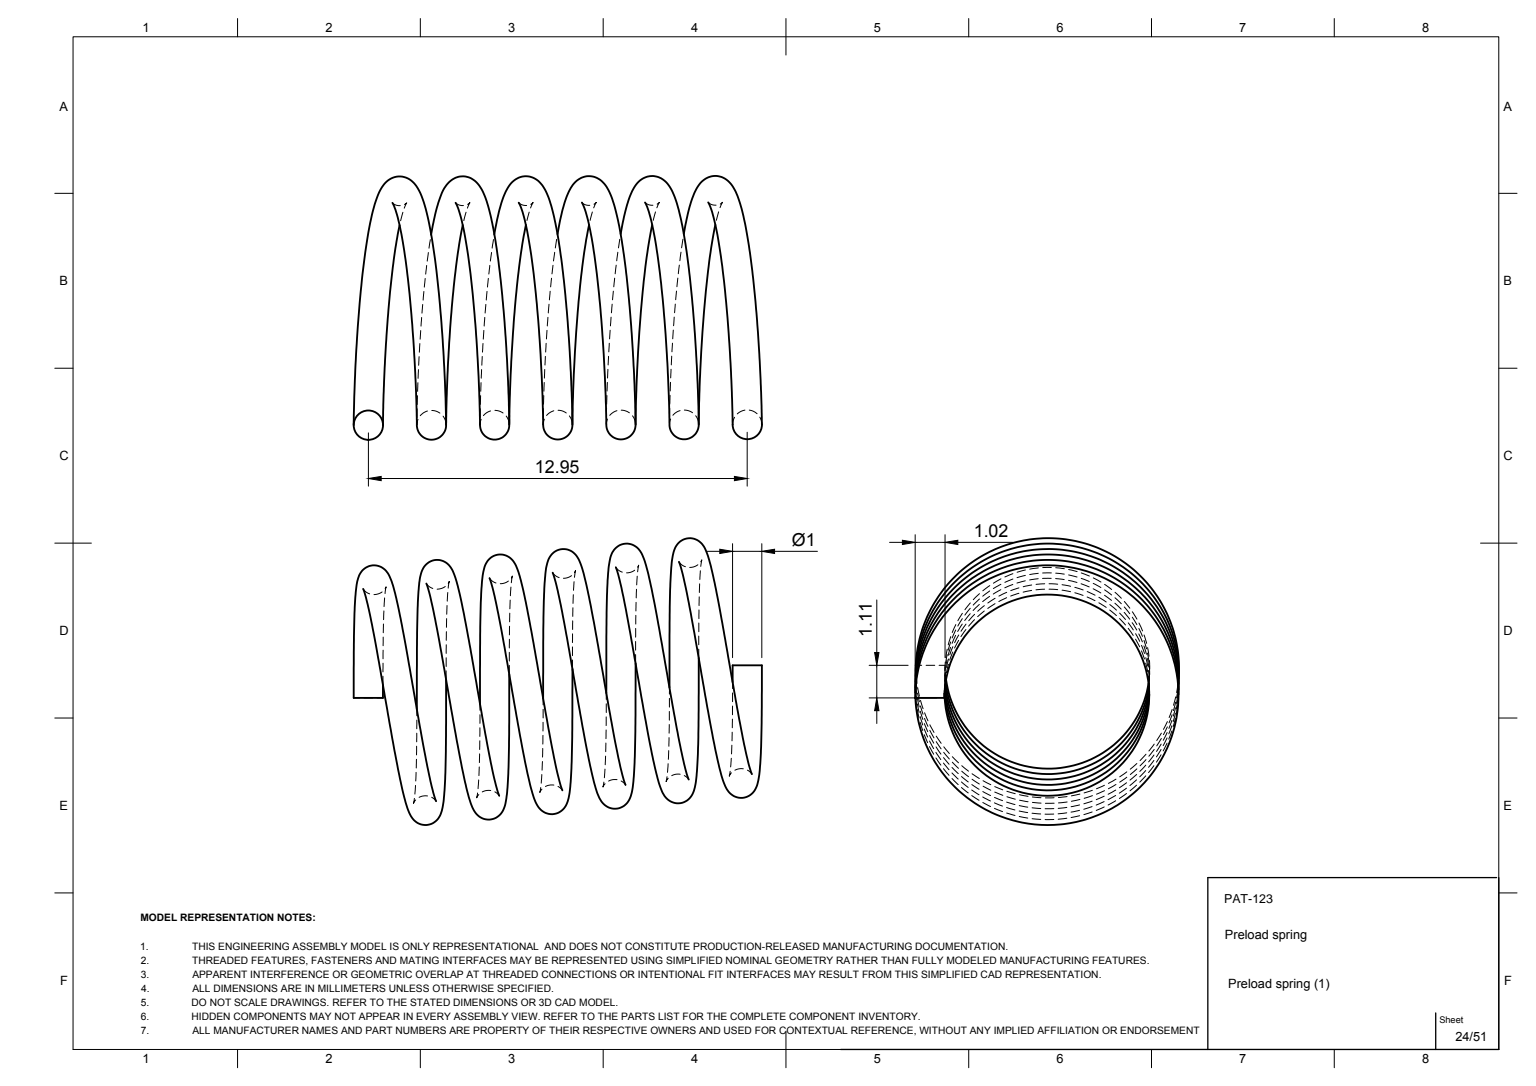
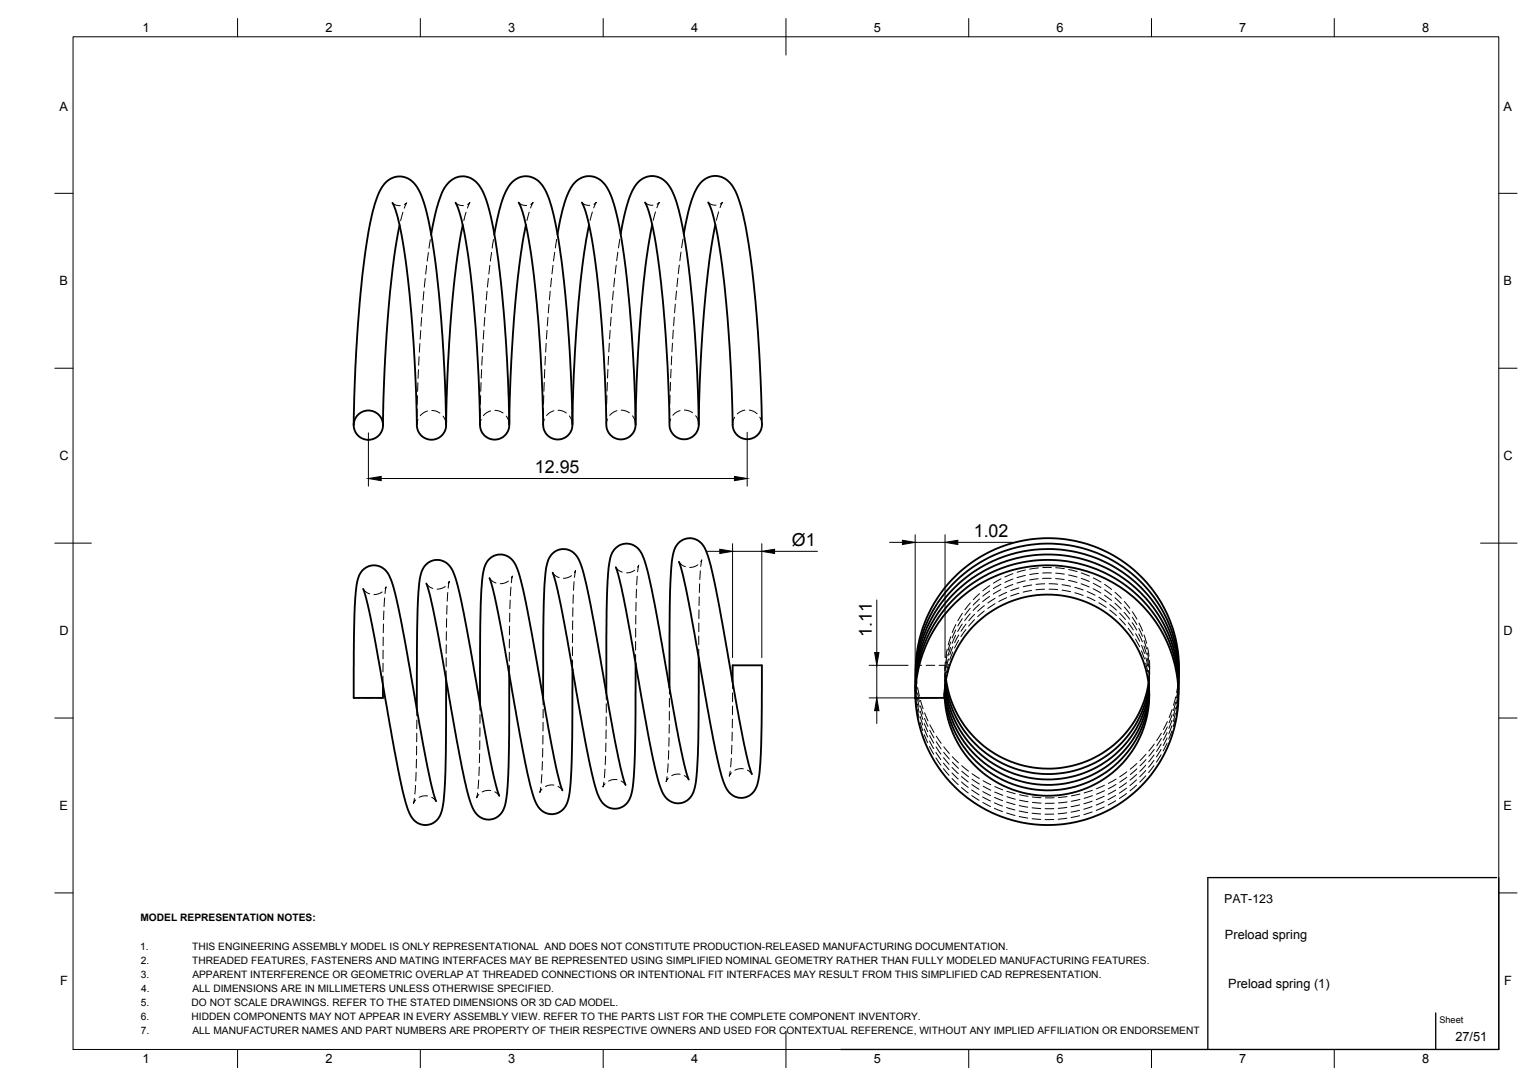
ISO-10303-21;
HEADER;
/* Generated by software containing ST-Developer
 * from STEP Tools, Inc. (www.steptools.com) 
 */

FILE_DESCRIPTION(
/* description */ ('Worm-less right-angle friction wheel drive'),
/* implementation_level */ '2;1');

FILE_NAME(
/* name */ 'Preload spring.step',
/* time_stamp */ '2026-10-28T03:22:36-07:00',
/* author */ (''),
/* organization */ (''),
/* preprocessor_version */ 'ST-DEVELOPER v20.2',
/* originating_system */ 'Autodesk Translation Framework v15.17.0.0',
/* authorisation */ '');

FILE_SCHEMA (('AUTOMOTIVE_DESIGN { 1 0 10303 214 3 1 1 }'));
ENDSEC;

DATA;
#10=MECHANICAL_DESIGN_GEOMETRIC_PRESENTATION_REPRESENTATION('',(#630),#17046);
#481=B_SPLINE_CURVE_WITH_KNOTS('',3,(#14322,#14323,#14324,#14325,#14326,
#14327,#14328,#14329,#14330,#14331,#14332,#14333,#14334,#14335,#14336,#14337,
#14338,#14339,#14340,#14341,#14342,#14343,#14344,#14345,#14346,#14347,#14348,
#14349,#14350,#14351,#14352,#14353,#14354,#14355,#14356,#14357,#14358,#14359,
#14360,#14361,#14362,#14363,#14364,#14365,#14366,#14367,#14368,#14369,#14370,
#14371,#14372,#14373,#14374,#14375,#14376,#14377,#14378,#14379,#14380,#14381,
#14382,#14383,#14384,#14385,#14386,#14387,#14388,#14389,#14390,#14391,#14392,
#14393,#14394,#14395,#14396,#14397,#14398,#14399,#14400,#14401,#14402,#14403,
#14404),.UNSPECIFIED.,.F.,.F.,(4,1,1,1,1,1,1,1,1,1,1,1,1,1,1,1,1,1,1,1,
1,1,1,1,1,1,1,1,1,1,1,1,1,1,1,1,1,1,1,1,1,1,1,1,1,1,1,1,1,1,1,1,1,1,1,1,
1,1,1,1,1,1,1,1,1,1,1,1,1,1,1,1,1,1,1,1,1,1,1,1,4),(0.,0.00892857142857143,
0.0178571428571429,0.0357142857142857,0.0535714285714286,0.0714285714285714,
0.0892857142857143,0.107142857142857,0.125,0.142857142857143,0.158730158730159,
0.174603174603175,0.19047619047619,0.202380952380952,0.214285714285714,
0.226190476190476,0.238095238095238,0.25,0.261904761904762,0.273809523809524,
0.285714285714286,0.297619047619048,0.30952380952381,0.321428571428571,
0.333333333333333,0.349206349206349,0.365079365079365,0.376984126984127,
0.380952380952381,0.392857142857143,0.404761904761905,0.416666666666667,
0.428571428571429,0.446428571428571,0.464285714285714,0.476190476190476,
0.488095238095238,0.5,0.508928571428571,0.517857142857143,0.526785714285714,
0.535714285714286,0.553571428571429,0.571428571428571,0.589285714285714,
0.607142857142857,0.625,0.633928571428571,0.642857142857143,0.654761904761905,
0.666666666666667,0.678571428571428,0.6875,0.696428571428571,0.705357142857143,
0.714285714285714,0.726190476190476,0.738095238095238,0.75,0.761904761904762,
0.773809523809524,0.785714285714286,0.791666666666667,0.797619047619047,
0.803571428571428,0.809523809523809,0.821428571428571,0.833333333333333,
0.845238095238095,0.857142857142857,0.866071428571429,0.875,0.883928571428571,
0.892857142857143,0.910714285714286,0.928571428571429,0.946428571428571,
0.964285714285714,0.982142857142857,0.991071428571429,1.),.UNSPECIFIED.);
#515=B_SPLINE_SURFACE_WITH_KNOTS('',3,3,((#13489,#13490,#13491,#13492,#13493,
#13494,#13495,#13496,#13497,#13498,#13499,#13500,#13501,#13502,#13503,#13504,
#13505,#13506,#13507,#13508,#13509,#13510,#13511,#13512,#13513,#13514,#13515,
#13516,#13517,#13518,#13519,#13520,#13521,#13522,#13523,#13524,#13525,#13526,
#13527,#13528,#13529,#13530,#13531,#13532,#13533,#13534,#13535,#13536,#13537,
#13538,#13539,#13540,#13541,#13542,#13543,#13544,#13545,#13546,#13547,#13548,
#13549,#13550,#13551,#13552,#13553,#13554,#13555,#13556,#13557,#13558,#13559,
#13560,#13561,#13562,#13563,#13564,#13565,#13566,#13567,#13568,#13569,#13570,
#13571),(#13572,#13573,#13574,#13575,#13576,#13577,#13578,#13579,#13580,
#13581,#13582,#13583,#13584,#13585,#13586,#13587,#13588,#13589,#13590,#13591,
#13592,#13593,#13594,#13595,#13596,#13597,#13598,#13599,#13600,#13601,#13602,
#13603,#13604,#13605,#13606,#13607,#13608,#13609,#13610,#13611,#13612,#13613,
#13614,#13615,#13616,#13617,#13618,#13619,#13620,#13621,#13622,#13623,#13624,
#13625,#13626,#13627,#13628,#13629,#13630,#13631,#13632,#13633,#13634,#13635,
#13636,#13637,#13638,#13639,#13640,#13641,#13642,#13643,#13644,#13645,#13646,
#13647,#13648,#13649,#13650,#13651,#13652,#13653,#13654),(#13655,#13656,
#13657,#13658,#13659,#13660,#13661,#13662,#13663,#13664,#13665,#13666,#13667,
#13668,#13669,#13670,#13671,#13672,#13673,#13674,#13675,#13676,#13677,#13678,
#13679,#13680,#13681,#13682,#13683,#13684,#13685,#13686,#13687,#13688,#13689,
#13690,#13691,#13692,#13693,#13694,#13695,#13696,#13697,#13698,#13699,#13700,
#13701,#13702,#13703,#13704,#13705,#13706,#13707,#13708,#13709,#13710,#13711,
#13712,#13713,#13714,#13715,#13716,#13717,#13718,#13719,#13720,#13721,#13722,
#13723,#13724,#13725,#13726,#13727,#13728,#13729,#13730,#13731,#13732,#13733,
#13734,#13735,#13736,#13737),(#13738,#13739,#13740,#13741,#13742,#13743,
#13744,#13745,#13746,#13747,#13748,#13749,#13750,#13751,#13752,#13753,#13754,
#13755,#13756,#13757,#13758,#13759,#13760,#13761,#13762,#13763,#13764,#13765,
#13766,#13767,#13768,#13769,#13770,#13771,#13772,#13773,#13774,#13775,#13776,
#13777,#13778,#13779,#13780,#13781,#13782,#13783,#13784,#13785,#13786,#13787,
#13788,#13789,#13790,#13791,#13792,#13793,#13794,#13795,#13796,#13797,#13798,
#13799,#13800,#13801,#13802,#13803,#13804,#13805,#13806,#13807,#13808,#13809,
#13810,#13811,#13812,#13813,#13814,#13815,#13816,#13817,#13818,#13819,#13820),
(#13821,#13822,#13823,#13824,#13825,#13826,#13827,#13828,#13829,#13830,
#13831,#13832,#13833,#13834,#13835,#13836,#13837,#13838,#13839,#13840,#13841,
#13842,#13843,#13844,#13845,#13846,#13847,#13848,#13849,#13850,#13851,#13852,
#13853,#13854,#13855,#13856,#13857,#13858,#13859,#13860,#13861,#13862,#13863,
#13864,#13865,#13866,#13867,#13868,#13869,#13870,#13871,#13872,#13873,#13874,
#13875,#13876,#13877,#13878,#13879,#13880,#13881,#13882,#13883,#13884,#13885,
#13886,#13887,#13888,#13889,#13890,#13891,#13892,#13893,#13894,#13895,#13896,
#13897,#13898,#13899,#13900,#13901,#13902,#13903),(#13904,#13905,#13906,
#13907,#13908,#13909,#13910,#13911,#13912,#13913,#13914,#13915,#13916,#13917,
#13918,#13919,#13920,#13921,#13922,#13923,#13924,#13925,#13926,#13927,#13928,
#13929,#13930,#13931,#13932,#13933,#13934,#13935,#13936,#13937,#13938,#13939,
#13940,#13941,#13942,#13943,#13944,#13945,#13946,#13947,#13948,#13949,#13950,
#13951,#13952,#13953,#13954,#13955,#13956,#13957,#13958,#13959,#13960,#13961,
#13962,#13963,#13964,#13965,#13966,#13967,#13968,#13969,#13970,#13971,#13972,
#13973,#13974,#13975,#13976,#13977,#13978,#13979,#13980,#13981,#13982,#13983,
#13984,#13985,#13986),(#13987,#13988,#13989,#13990,#13991,#13992,#13993,
#13994,#13995,#13996,#13997,#13998,#13999,#14000,#14001,#14002,#14003,#14004,
#14005,#14006,#14007,#14008,#14009,#14010,#14011,#14012,#14013,#14014,#14015,
#14016,#14017,#14018,#14019,#14020,#14021,#14022,#14023,#14024,#14025,#14026,
#14027,#14028,#14029,#14030,#14031,#14032,#14033,#14034,#14035,#14036,#14037,
#14038,#14039,#14040,#14041,#14042,#14043,#14044,#14045,#14046,#14047,#14048,
#14049,#14050,#14051,#14052,#14053,#14054,#14055,#14056,#14057,#14058,#14059,
#14060,#14061,#14062,#14063,#14064,#14065,#14066,#14067,#14068,#14069),
(#14070,#14071,#14072,#14073,#14074,#14075,#14076,#14077,#14078,#14079,
#14080,#14081,#14082,#14083,#14084,#14085,#14086,#14087,#14088,#14089,#14090,
#14091,#14092,#14093,#14094,#14095,#14096,#14097,#14098,#14099,#14100,#14101,
#14102,#14103,#14104,#14105,#14106,#14107,#14108,#14109,#14110,#14111,#14112,
#14113,#14114,#14115,#14116,#14117,#14118,#14119,#14120,#14121,#14122,#14123,
#14124,#14125,#14126,#14127,#14128,#14129,#14130,#14131,#14132,#14133,#14134,
#14135,#14136,#14137,#14138,#14139,#14140,#14141,#14142,#14143,#14144,#14145,
#14146,#14147,#14148,#14149,#14150,#14151,#14152),(#14153,#14154,#14155,
#14156,#14157,#14158,#14159,#14160,#14161,#14162,#14163,#14164,#14165,#14166,
#14167,#14168,#14169,#14170,#14171,#14172,#14173,#14174,#14175,#14176,#14177,
#14178,#14179,#14180,#14181,#14182,#14183,#14184,#14185,#14186,#14187,#14188,
#14189,#14190,#14191,#14192,#14193,#14194,#14195,#14196,#14197,#14198,#14199,
#14200,#14201,#14202,#14203,#14204,#14205,#14206,#14207,#14208,#14209,#14210,
#14211,#14212,#14213,#14214,#14215,#14216,#14217,#14218,#14219,#14220,#14221,
#14222,#14223,#14224,#14225,#14226,#14227,#14228,#14229,#14230,#14231,#14232,
#14233,#14234,#14235),(#14236,#14237,#14238,#14239,#14240,#14241,#14242,
#14243,#14244,#14245,#14246,#14247,#14248,#14249,#14250,#14251,#14252,#14253,
#14254,#14255,#14256,#14257,#14258,#14259,#14260,#14261,#14262,#14263,#14264,
#14265,#14266,#14267,#14268,#14269,#14270,#14271,#14272,#14273,#14274,#14275,
#14276,#14277,#14278,#14279,#14280,#14281,#14282,#14283,#14284,#14285,#14286,
#14287,#14288,#14289,#14290,#14291,#14292,#14293,#14294,#14295,#14296,#14297,
#14298,#14299,#14300,#14301,#14302,#14303,#14304,#14305,#14306,#14307,#14308,
#14309,#14310,#14311,#14312,#14313,#14314,#14315,#14316,#14317,#14318)),
 .UNSPECIFIED.,.T.,.F.,.F.,(4,1,1,1,1,1,1,4),(4,1,1,1,1,1,1,1,1,1,1,1,1,
1,1,1,1,1,1,1,1,1,1,1,1,1,1,1,1,1,1,1,1,1,1,1,1,1,1,1,1,1,1,1,1,1,1,1,1,
1,1,1,1,1,1,1,1,1,1,1,1,1,1,1,1,1,1,1,1,1,1,1,1,1,1,1,1,1,1,1,4),(-3.14159265358979,
-2.24399475256414,-1.34639685153848,-0.448798950512828,0.448798950512828,
1.34639685153848,2.24399475256414,3.14159265358979),(0.,0.00892857142857143,
0.0178571428571429,0.0357142857142857,0.0535714285714286,0.0714285714285714,
0.0892857142857143,0.107142857142857,0.125,0.142857142857143,0.158730158730159,
0.174603174603175,0.19047619047619,0.202380952380952,0.214285714285714,
0.226190476190476,0.238095238095238,0.25,0.261904761904762,0.273809523809524,
0.285714285714286,0.297619047619048,0.30952380952381,0.321428571428571,
0.333333333333333,0.349206349206349,0.365079365079365,0.376984126984127,
0.380952380952381,0.392857142857143,0.404761904761905,0.416666666666667,
0.428571428571429,0.446428571428571,0.464285714285714,0.476190476190476,
0.488095238095238,0.5,0.508928571428571,0.517857142857143,0.526785714285714,
0.535714285714286,0.553571428571429,0.571428571428571,0.589285714285714,
0.607142857142857,0.625,0.633928571428571,0.642857142857143,0.654761904761905,
0.666666666666667,0.678571428571428,0.6875,0.696428571428571,0.705357142857143,
0.714285714285714,0.726190476190476,0.738095238095238,0.75,0.761904761904762,
0.773809523809524,0.785714285714286,0.791666666666667,0.797619047619047,
0.803571428571428,0.809523809523809,0.821428571428571,0.833333333333333,
0.845238095238095,0.857142857142857,0.866071428571429,0.875,0.883928571428571,
0.892857142857143,0.910714285714286,0.928571428571429,0.946428571428571,
0.964285714285714,0.982142857142857,0.991071428571429,1.),.UNSPECIFIED.);
#536=SHAPE_REPRESENTATION_RELATIONSHIP('SRR','None',#17279,#583);
#583=ADVANCED_BREP_SHAPE_REPRESENTATION('',(#684),#17015);
#630=STYLED_ITEM('',(#17591),#684);
#684=MANIFOLD_SOLID_BREP('Body1',#8185);
#1060=PLANE('',#9216);
#1061=PLANE('',#9217);
#1430=FACE_OUTER_BOUND('',#2086,.T.);
#1431=FACE_OUTER_BOUND('',#2087,.T.);
#1432=FACE_OUTER_BOUND('',#2088,.T.);
#2086=EDGE_LOOP('',(#6578,#6579,#6580,#6581));
#2087=EDGE_LOOP('',(#6582));
#2088=EDGE_LOOP('',(#6583));
#3685=CIRCLE('',#9214,0.05);
#3686=CIRCLE('',#9215,0.05);
#4217=VERTEX_POINT('',#14319);
#4218=VERTEX_POINT('',#14321);
#5058=EDGE_CURVE('',#4217,#4217,#3685,.T.);
#5059=EDGE_CURVE('',#4217,#4218,#481,.T.);
#5060=EDGE_CURVE('',#4218,#4218,#3686,.T.);
#6578=ORIENTED_EDGE('',*,*,#5058,.T.);
#6579=ORIENTED_EDGE('',*,*,#5059,.T.);
#6580=ORIENTED_EDGE('',*,*,#5060,.F.);
#6581=ORIENTED_EDGE('',*,*,#5059,.F.);
#6582=ORIENTED_EDGE('',*,*,#5060,.T.);
#6583=ORIENTED_EDGE('',*,*,#5058,.F.);
#7922=ADVANCED_FACE('',(#1430),#515,.T.);
#7923=ADVANCED_FACE('',(#1431),#1060,.T.);
#7924=ADVANCED_FACE('',(#1432),#1061,.F.);
#8185=CLOSED_SHELL('',(#7922,#7923,#7924));
#9213=AXIS2_PLACEMENT_3D('',#13488,#11009,#11010);
#9214=AXIS2_PLACEMENT_3D('',#14320,#11011,#11012);
#9215=AXIS2_PLACEMENT_3D('',#14405,#11013,#11014);
#9216=AXIS2_PLACEMENT_3D('',#14406,#11015,#11016);
#9217=AXIS2_PLACEMENT_3D('',#14407,#11017,#11018);
#11009=DIRECTION('axis',(0.,0.,1.));
#11010=DIRECTION('refdir',(1.,0.,0.));
#11011=DIRECTION('center_axis',(-0.000134420183300025,-0.085636011539688,
0.996326480356107));
#11012=DIRECTION('ref_axis',(1.1553650826854E-5,-0.996326489423811,-0.0856360107603029));
#11013=DIRECTION('center_axis',(0.000134419999317792,-0.085636011399563,
0.996326480368176));
#11014=DIRECTION('ref_axis',(0.0962365814952688,0.991703136101715,0.0852256430197378));
#11015=DIRECTION('center_axis',(0.000134419999317792,-0.085636011399563,
0.996326480368176));
#11016=DIRECTION('ref_axis',(0.0962365814952688,0.991703136101715,0.0852256430197378));
#11017=DIRECTION('center_axis',(-0.000134420183300025,-0.085636011539688,
0.996326480356107));
#11018=DIRECTION('ref_axis',(1.1553650826854E-5,-0.996326489423811,-0.0856360107603029));
#13488=CARTESIAN_POINT('',(0.,0.,0.));
#13489=CARTESIAN_POINT('Ctrl Pts',(0.0999994223174587,7.09981632447119,
4.00428180053801));
#13490=CARTESIAN_POINT('Ctrl Pts',(0.0999933436797077,7.09594376396835,
4.04933684813297));
#13491=CARTESIAN_POINT('Ctrl Pts',(0.0846594327171957,7.08819408394972,
4.13908992957458));
#13492=CARTESIAN_POINT('Ctrl Pts',(-0.00357043069494361,7.07263318914228,
4.29963340285418));
#13493=CARTESIAN_POINT('Ctrl Pts',(-0.206356294917572,7.05308143195573,
4.42766373470968));
#13494=CARTESIAN_POINT('Ctrl Pts',(-0.494863120131574,7.02945164505109,
4.39548903188326));
#13495=CARTESIAN_POINT('Ctrl Pts',(-0.701612481834811,7.00565862484048,
4.18915927264886));
#13496=CARTESIAN_POINT('Ctrl Pts',(-0.734902354617378,6.98170298771966,
3.89687986754614));
#13497=CARTESIAN_POINT('Ctrl Pts',(-0.577665286755769,6.9575878275568,3.64601239877861));
#13498=CARTESIAN_POINT('Ctrl Pts',(-0.296425446296891,6.93331589731144,
3.54721069783272));
#13499=CARTESIAN_POINT('Ctrl Pts',(-0.0238970429973844,6.90979548741706,
3.64245102870328));
#13500=CARTESIAN_POINT('Ctrl Pts',(0.131586191166419,6.88704931445005,3.8704985271515));
#13501=CARTESIAN_POINT('Ctrl Pts',(0.132036205657411,6.86509836852865,4.13674945418924));
#13502=CARTESIAN_POINT('Ctrl Pts',(-0.0060413687179679,6.84487478558125,
4.33958298894643));
#13503=CARTESIAN_POINT('Ctrl Pts',(-0.204116844890033,6.82641141958407,
4.43475944317313));
#13504=CARTESIAN_POINT('Ctrl Pts',(-0.402473369433673,6.80973569344043,
4.43486896119673));
#13505=CARTESIAN_POINT('Ctrl Pts',(-0.581827228221285,6.79300305116116,
4.34852221416367));
#13506=CARTESIAN_POINT('Ctrl Pts',(-0.706454134874152,6.7762153628094,4.192464816352));
#13507=CARTESIAN_POINT('Ctrl Pts',(-0.751016294559626,6.75937457420164,
3.99715087739011));
#13508=CARTESIAN_POINT('Ctrl Pts',(-0.706447662037028,6.74248271608976,
3.80123388795173));
#13509=CARTESIAN_POINT('Ctrl Pts',(-0.580873534358325,6.72554188917784,
3.64359934962882));
#13510=CARTESIAN_POINT('Ctrl Pts',(-0.398793807750649,6.70855427056295,
3.55588854173989));
#13511=CARTESIAN_POINT('Ctrl Pts',(-0.196213186746174,6.69152210478501,
3.55582569363604));
#13512=CARTESIAN_POINT('Ctrl Pts',(-0.0130963934752721,6.67444770586136,
3.64392728654252));
#13513=CARTESIAN_POINT('Ctrl Pts',(0.113707820363769,6.65733344528682,3.80305624025719));
#13514=CARTESIAN_POINT('Ctrl Pts',(0.164656362590817,6.63827601697293,4.02413741573514));
#13515=CARTESIAN_POINT('Ctrl Pts',(0.0896082709820025,6.61726302509207,
4.2676978223342));
#13516=CARTESIAN_POINT('Ctrl Pts',(-0.110245732077343,6.59619863179822,
4.4270642600818));
#13517=CARTESIAN_POINT('Ctrl Pts',(-0.290838098938005,6.58084997747224,
4.45395573001046));
#13518=CARTESIAN_POINT('Ctrl Pts',(-0.445467117475853,6.56740673782488,
4.43069910759464));
#13519=CARTESIAN_POINT('Ctrl Pts',(-0.589663880409842,6.55395079532829,
4.36131796304211));
#13520=CARTESIAN_POINT('Ctrl Pts',(-0.718225707768932,6.53662851071928,
4.20020661739991));
#13521=CARTESIAN_POINT('Ctrl Pts',(-0.763898158866166,6.51928717897976,
3.99912848715837));
#13522=CARTESIAN_POINT('Ctrl Pts',(-0.710721419612997,6.49903664059857,
3.764202830041));
#13523=CARTESIAN_POINT('Ctrl Pts',(-0.510149997687367,6.47587070043553,
3.56253207697483));
#13524=CARTESIAN_POINT('Ctrl Pts',(-0.227250362890276,6.45268625633124,
3.53107252428385));
#13525=CARTESIAN_POINT('Ctrl Pts',(-0.00982453983942397,6.43239259089565,
3.63631313688574));
#13526=CARTESIAN_POINT('Ctrl Pts',(0.119224416062016,6.414995879623,3.79796488057796));
#13527=CARTESIAN_POINT('Ctrl Pts',(0.161414220224748,6.39904954972701,3.98302626625864));
#13528=CARTESIAN_POINT('Ctrl Pts',(0.132781651753175,6.38455548538367,4.15109736344141));
#13529=CARTESIAN_POINT('Ctrl Pts',(0.058591217696994,6.37151403493753,4.28547086198332));
#13530=CARTESIAN_POINT('Ctrl Pts',(-0.0558362639783319,6.35847699034469,
4.38747481451575));
#13531=CARTESIAN_POINT('Ctrl Pts',(-0.244624220570673,6.34110173177432,
4.46620946091905));
#13532=CARTESIAN_POINT('Ctrl Pts',(-0.509258386493358,6.31939963958705,
4.43663450707748));
#13533=CARTESIAN_POINT('Ctrl Pts',(-0.735030443095589,6.29339375292805,
4.21063569075453));
#13534=CARTESIAN_POINT('Ctrl Pts',(-0.770492148406669,6.2674338232997,3.89395438143295));
#13535=CARTESIAN_POINT('Ctrl Pts',(-0.601210048531917,6.24152902186401,
3.62457992816658));
#13536=CARTESIAN_POINT('Ctrl Pts',(-0.351688619951789,6.21999512440529,
3.53770552245775));
#13537=CARTESIAN_POINT('Ctrl Pts',(-0.152299417857812,6.20280445728418,
3.57207084012085));
#13538=CARTESIAN_POINT('Ctrl Pts',(-0.00495835013055459,6.18850033974624,
3.65330634586973));
#13539=CARTESIAN_POINT('Ctrl Pts',(0.111522803781729,6.17279483671223,3.79940640678234));
#13540=CARTESIAN_POINT('Ctrl Pts',(0.156701474788417,6.15570021231953,3.99770463755195));
#13541=CARTESIAN_POINT('Ctrl Pts',(0.115262604711903,6.14006777305336,4.17897821875209));
#13542=CARTESIAN_POINT('Ctrl Pts',(0.0185932180471106,6.12588811043834,
4.31497113433199));
#13543=CARTESIAN_POINT('Ctrl Pts',(-0.103590553659916,6.11315178814851,
4.4016989608744));
#13544=CARTESIAN_POINT('Ctrl Pts',(-0.247293954733903,6.1004417858412,4.44304193852122));
#13545=CARTESIAN_POINT('Ctrl Pts',(-0.412869049658234,6.08634982725544,
4.43379507168706));
#13546=CARTESIAN_POINT('Ctrl Pts',(-0.578482300908516,6.07088880084204,
4.3539190346138));
#13547=CARTESIAN_POINT('Ctrl Pts',(-0.703246723757797,6.05407432044984,
4.19753682982269));
#13548=CARTESIAN_POINT('Ctrl Pts',(-0.747469580607062,6.03731392465469,
4.00314057125818));
#13549=CARTESIAN_POINT('Ctrl Pts',(-0.703238625925696,6.02060951959296,
3.80940575329504));
#13550=CARTESIAN_POINT('Ctrl Pts',(-0.579634776479789,6.00396293095479,
3.65467865258803));
#13551=CARTESIAN_POINT('Ctrl Pts',(-0.431500759601328,5.99014040360805,
3.58338254073736));
#13552=CARTESIAN_POINT('Ctrl Pts',(-0.303561319206374,5.97911298339926,
3.56906449106088));
#13553=CARTESIAN_POINT('Ctrl Pts',(-0.207808748835976,5.97085791464426,
3.57983145987356));
#13554=CARTESIAN_POINT('Ctrl Pts',(-0.117044922248722,5.96261853714979,
3.6116348383249));
#13555=CARTESIAN_POINT('Ctrl Pts',(-0.00861997369778145,5.95165386736835,
3.67968231581426));
#13556=CARTESIAN_POINT('Ctrl Pts',(0.0926329081004657,5.93798817658918,
3.80681756846826));
#13557=CARTESIAN_POINT('Ctrl Pts',(0.135870644163702,5.92165495155963,3.99626375633351));
#13558=CARTESIAN_POINT('Ctrl Pts',(0.0926387969430078,5.90538860209907,
4.18487776410349));
#13559=CARTESIAN_POINT('Ctrl Pts',(-0.0175125738479973,5.89054016294629,
4.32293582509909));
#13560=CARTESIAN_POINT('Ctrl Pts',(-0.156061008534171,5.87709197920747,
4.39936287338782));
#13561=CARTESIAN_POINT('Ctrl Pts',(-0.296018497756522,5.86502791432804,
4.42315611503599));
#13562=CARTESIAN_POINT('Ctrl Pts',(-0.435406476921251,5.8530035361086,4.39932451423293));
#13563=CARTESIAN_POINT('Ctrl Pts',(-0.600212844195293,5.83702437044493,
4.30861645270809));
#13564=CARTESIAN_POINT('Ctrl Pts',(-0.729945333339283,5.81715142573852,
4.10216892170714));
#13565=CARTESIAN_POINT('Ctrl Pts',(-0.696976009348358,5.7934671926544,3.81306008549607));
#13566=CARTESIAN_POINT('Ctrl Pts',(-0.492652698548329,5.76994854996481,
3.60918617550531));
#13567=CARTESIAN_POINT('Ctrl Pts',(-0.207515825799976,5.74659510021081,
3.57736699868709));
#13568=CARTESIAN_POINT('Ctrl Pts',(-0.00714719245692835,5.72727465695078,
3.70390131122158));
#13569=CARTESIAN_POINT('Ctrl Pts',(0.0800330609517386,5.71189866882786,
3.86253474741929));
#13570=CARTESIAN_POINT('Ctrl Pts',(0.0951821641861108,5.70424160396714,
3.95121652410011));
#13571=CARTESIAN_POINT('Ctrl Pts',(0.0951881709252366,5.70041484319491,
3.99573871784903));
#13572=CARTESIAN_POINT('Ctrl Pts',(0.0850394574365172,7.09981632447119,
4.00427978220239));
#13573=CARTESIAN_POINT('Ctrl Pts',(0.0850336018816217,7.09608588493208,
4.04768133289773));
#13574=CARTESIAN_POINT('Ctrl Pts',(0.0702699903358584,7.08862397630483,
4.1341064684711));
#13575=CARTESIAN_POINT('Ctrl Pts',(-0.0147069746650678,7.07363615104764,
4.28874312195255));
#13576=CARTESIAN_POINT('Ctrl Pts',(-0.210062520100004,7.05480250014203,
4.4121050616425));
#13577=CARTESIAN_POINT('Ctrl Pts',(-0.488174822436898,7.03202630176359,
4.38112095270672));
#13578=CARTESIAN_POINT('Ctrl Pts',(-0.687626117343361,7.0090788623615,4.18212006759028));
#13579=CARTESIAN_POINT('Ctrl Pts',(-0.719801750366849,6.98595686154072,
3.89998017636458));
#13580=CARTESIAN_POINT('Ctrl Pts',(-0.567925280966783,6.9626613445872,3.65757702153162));
#13581=CARTESIAN_POINT('Ctrl Pts',(-0.295960145703228,6.93919201998295,
3.56197635348132));
#13582=CARTESIAN_POINT('Ctrl Pts',(-0.0321049966673812,6.91642613922016,
3.65412444008679));
#13583=CARTESIAN_POINT('Ctrl Pts',(0.118620874938022,6.89438553806723,3.87511047955543));
#13584=CARTESIAN_POINT('Ctrl Pts',(0.119105685200114,6.87309055560467,4.13343111127147));
#13585=CARTESIAN_POINT('Ctrl Pts',(-0.0149725090072682,6.85345021204612,
4.33047273617547));
#13586=CARTESIAN_POINT('Ctrl Pts',(-0.207553265723982,6.83550152476108,
4.42303755552263));
#13587=CARTESIAN_POINT('Ctrl Pts',(-0.400605820874248,6.81927426099695,
4.42316739110795));
#13588=CARTESIAN_POINT('Ctrl Pts',(-0.575349585461221,6.80297292453282,
4.3390616393177));
#13589=CARTESIAN_POINT('Ctrl Pts',(-0.696901935083712,6.78660524474866,
4.18689685110264));
#13590=CARTESIAN_POINT('Ctrl Pts',(-0.740422898887374,6.77016837055957,
3.99624089239393));
#13591=CARTESIAN_POINT('Ctrl Pts',(-0.696895127946879,6.75366348159961,
3.80478155122518));
#13592=CARTESIAN_POINT('Ctrl Pts',(-0.57406933450842,6.73709380592631,3.65055798081225));
#13593=CARTESIAN_POINT('Ctrl Pts',(-0.395769076508023,6.72046256251377,
3.56463827820055));
#13594=CARTESIAN_POINT('Ctrl Pts',(-0.197154892631745,6.70376777233271,
3.56455003028145));
#13595=CARTESIAN_POINT('Ctrl Pts',(-0.0174072167564555,6.68701354119935,
3.65099852210416));
#13596=CARTESIAN_POINT('Ctrl Pts',(0.107219695584159,6.67019963849409,3.80735503098315));
#13597=CARTESIAN_POINT('Ctrl Pts',(0.157377024534706,6.65145770741293,4.02484224001632));
#13598=CARTESIAN_POINT('Ctrl Pts',(0.0834907936109698,6.63075558432489,
4.26482879249461));
#13599=CARTESIAN_POINT('Ctrl Pts',(-0.113676877997255,6.60997502326179,
4.4221382080455));
#13600=CARTESIAN_POINT('Ctrl Pts',(-0.292136244859537,6.5948103064137,4.44873719553528));
#13601=CARTESIAN_POINT('Ctrl Pts',(-0.445072347899979,6.58151560551988,
4.42573828157157));
#13602=CARTESIAN_POINT('Ctrl Pts',(-0.587808705388691,6.56819972291512,
4.35708244751097));
#13603=CARTESIAN_POINT('Ctrl Pts',(-0.715254356693917,6.55103194356631,
4.19742039979326));
#13604=CARTESIAN_POINT('Ctrl Pts',(-0.760601355295959,6.53382909817788,
3.99789591592248));
#13605=CARTESIAN_POINT('Ctrl Pts',(-0.7078026422373,6.51371065102388,3.76447139208622));
#13606=CARTESIAN_POINT('Ctrl Pts',(-0.508287882172965,6.49066883804046,
3.56373316987723));
#13607=CARTESIAN_POINT('Ctrl Pts',(-0.226234240731051,6.46755740591608,
3.53227686762576));
#13608=CARTESIAN_POINT('Ctrl Pts',(-0.00909244890320504,6.44729795655168,
3.63734053951694));
#13609=CARTESIAN_POINT('Ctrl Pts',(0.119970850340226,6.42990267527582,3.79896825205898));
#13610=CARTESIAN_POINT('Ctrl Pts',(0.162236447406711,6.41394240449883,3.98423317997473));
#13611=CARTESIAN_POINT('Ctrl Pts',(0.133549532561585,6.39941634657213,4.15269512343536));
#13612=CARTESIAN_POINT('Ctrl Pts',(0.059128979758546,6.38633399253393,4.28751171624146));
#13613=CARTESIAN_POINT('Ctrl Pts',(-0.0557735754439485,6.37324413074094,
4.38995105707331));
#13614=CARTESIAN_POINT('Ctrl Pts',(-0.245522966737918,6.35578135522631,
4.46910560844112));
#13615=CARTESIAN_POINT('Ctrl Pts',(-0.511891841221142,6.33394317857852,
4.43941437761895));
#13616=CARTESIAN_POINT('Ctrl Pts',(-0.73964230083353,6.30772004879476,4.21157475252753));
#13617=CARTESIAN_POINT('Ctrl Pts',(-0.775562357309942,6.28150419722604,
3.89165585318146));
#13618=CARTESIAN_POINT('Ctrl Pts',(-0.604311957412975,6.25529235214756,
3.61896952975546));
#13619=CARTESIAN_POINT('Ctrl Pts',(-0.351351084360445,6.23346807877194,
3.53081646027971));
#13620=CARTESIAN_POINT('Ctrl Pts',(-0.148911855072523,6.21601731725428,
3.56569131592939));
#13621=CARTESIAN_POINT('Ctrl Pts',(0.000808738546099167,6.20148503609852,
3.64822598806359));
#13622=CARTESIAN_POINT('Ctrl Pts',(0.119307888319452,6.18551200572715,3.79681481925343));
#13623=CARTESIAN_POINT('Ctrl Pts',(0.165336825909723,6.16810621199183,3.99873450926149));
#13624=CARTESIAN_POINT('Ctrl Pts',(0.12311936738889,6.15217178129263,4.1835309684545));
#13625=CARTESIAN_POINT('Ctrl Pts',(0.024491947298141,6.13770537799267,4.32229762424903));
#13626=CARTESIAN_POINT('Ctrl Pts',(-0.10026800379765,6.12470150020605,4.41086793897621));
#13627=CARTESIAN_POINT('Ctrl Pts',(-0.247118546887194,6.1117152886378,4.45312483699181));
#13628=CARTESIAN_POINT('Ctrl Pts',(-0.416459720890053,6.09730438243501,
4.44367875235149));
#13629=CARTESIAN_POINT('Ctrl Pts',(-0.585994266630716,6.08147960761965,
4.36192882635867));
#13630=CARTESIAN_POINT('Ctrl Pts',(-0.71384850238361,6.06425381154321,4.20171116423524));
#13631=CARTESIAN_POINT('Ctrl Pts',(-0.759222000808869,6.04706459967159,
4.00233367493855));
#13632=CARTESIAN_POINT('Ctrl Pts',(-0.713838394267311,6.02991914561157,
3.80345284952215));
#13633=CARTESIAN_POINT('Ctrl Pts',(-0.58685029737105,6.01281745749491,3.64446602567488));
#13634=CARTESIAN_POINT('Ctrl Pts',(-0.434523741076119,5.99860459894777,
3.57113647661554));
#13635=CARTESIAN_POINT('Ctrl Pts',(-0.302871593009492,5.98725781105221,
3.55640154880377));
#13636=CARTESIAN_POINT('Ctrl Pts',(-0.204299994389332,5.97875983751493,
3.56748322724138));
#13637=CARTESIAN_POINT('Ctrl Pts',(-0.110827457753729,5.97027500248914,
3.60023416597451));
#13638=CARTESIAN_POINT('Ctrl Pts',(0.000877339158924813,5.95897911565719,
3.67033627955141));
#13639=CARTESIAN_POINT('Ctrl Pts',(0.105257286966471,5.94489365179489,3.80137990843985));
#13640=CARTESIAN_POINT('Ctrl Pts',(0.149873797036135,5.92804610367806,3.99679794750918));
#13641=CARTESIAN_POINT('Ctrl Pts',(0.105257359738255,5.91125630747322,4.19149770579706));
#13642=CARTESIAN_POINT('Ctrl Pts',(-0.00851130012522223,5.89591960107197,
4.33410736914532));
#13643=CARTESIAN_POINT('Ctrl Pts',(-0.151696220437804,5.88202155769958,
4.41309722089718));
#13644=CARTESIAN_POINT('Ctrl Pts',(-0.296398986774869,5.86954879341379,
4.43770080209349));
#13645=CARTESIAN_POINT('Ctrl Pts',(-0.440573237144837,5.85711192694754,
4.41305386836028));
#13646=CARTESIAN_POINT('Ctrl Pts',(-0.611104421885485,5.84057809075553,
4.31920084666369));
#13647=CARTESIAN_POINT('Ctrl Pts',(-0.745431119265092,5.82000461576502,
4.10548372373842));
#13648=CARTESIAN_POINT('Ctrl Pts',(-0.711300999956552,5.79546993853416,
3.80598914689769));
#13649=CARTESIAN_POINT('Ctrl Pts',(-0.499541348546689,5.77109407410407,
3.59467599283417));
#13650=CARTESIAN_POINT('Ctrl Pts',(-0.203895328638292,5.7468798977641,3.56167095656836));
#13651=CARTESIAN_POINT('Ctrl Pts',(0.00392749184947024,5.72684068907964,
3.6929091997083));
#13652=CARTESIAN_POINT('Ctrl Pts',(0.0943564738679285,5.7108922189658,3.85744827453292));
#13653=CARTESIAN_POINT('Ctrl Pts',(0.110072470175732,5.70294882509164,3.94944546934011));
#13654=CARTESIAN_POINT('Ctrl Pts',(0.110078698955025,5.69898060743533,3.99561343380099));
#13655=CARTESIAN_POINT('Ctrl Pts',(0.0552109446983192,7.08554097311938,
4.00304876633418));
#13656=CARTESIAN_POINT('Ctrl Pts',(0.0552055358490416,7.08209511947001,
4.04313932142398));
#13657=CARTESIAN_POINT('Ctrl Pts',(0.0415778810591391,7.07520994153035,
4.12288334405912));
#13658=CARTESIAN_POINT('Ctrl Pts',(-0.0367895863384045,7.06138952221764,
4.26547075358216));
#13659=CARTESIAN_POINT('Ctrl Pts',(-0.216751774778633,7.04404262129843,
4.37904913409819));
#13660=CARTESIAN_POINT('Ctrl Pts',(-0.472633848843551,7.0230861784788,4.35049327462187));
#13661=CARTESIAN_POINT('Ctrl Pts',(-0.655980880788529,7.00198852558813,
4.16750943496815));
#13662=CARTESIAN_POINT('Ctrl Pts',(-0.685529083724197,6.98073994105562,
3.90823429417137));
#13663=CARTESIAN_POINT('Ctrl Pts',(-0.545981564425269,6.95933520737526,
3.68551901603162));
#13664=CARTESIAN_POINT('Ctrl Pts',(-0.296075489511932,6.93776772965475,
3.59766361550569));
#13665=CARTESIAN_POINT('Ctrl Pts',(-0.0535123959286835,6.91683750495745,
3.68235541997892));
#13666=CARTESIAN_POINT('Ctrl Pts',(0.0851561523655047,6.89656078808882,
3.88562267842967));
#13667=CARTESIAN_POINT('Ctrl Pts',(0.0856311510431353,6.87695461538451,
4.12343923801433));
#13668=CARTESIAN_POINT('Ctrl Pts',(-0.037907049429957,6.85885216444035,
4.30504970436046));
#13669=CARTESIAN_POINT('Ctrl Pts',(-0.215577868848402,6.84229013135253,
4.3904699811323));
#13670=CARTESIAN_POINT('Ctrl Pts',(-0.393871042935876,6.82730164024858,
4.39060863287945));
#13671=CARTESIAN_POINT('Ctrl Pts',(-0.555445579066094,6.81222960735315,
4.31286947512227));
#13672=CARTESIAN_POINT('Ctrl Pts',(-0.667991397971185,6.7970745501898,4.17201470408707));
#13673=CARTESIAN_POINT('Ctrl Pts',(-0.708363930243454,6.78183538373591,
3.99528088580219));
#13674=CARTESIAN_POINT('Ctrl Pts',(-0.667982499492249,6.76651159301788,
3.8175383544735));
#13675=CARTESIAN_POINT('Ctrl Pts',(-0.553809065445986,6.75110329506063,
3.67412832553629));
#13676=CARTESIAN_POINT('Ctrl Pts',(-0.387770718002321,6.73561041405154,
3.59408217536656));
#13677=CARTESIAN_POINT('Ctrl Pts',(-0.202486939836806,6.72003270044929,
3.59396650356072));
#13678=CARTESIAN_POINT('Ctrl Pts',(-0.0344849723331165,6.70437042642184,
3.67472585533919));
#13679=CARTESIAN_POINT('Ctrl Pts',(0.0822359686491668,6.6886238248135,3.82110359305832));
#13680=CARTESIAN_POINT('Ctrl Pts',(0.129333318074877,6.6710343619389,4.02513087435611));
#13681=CARTESIAN_POINT('Ctrl Pts',(0.0599513621413444,6.65156705091096,
4.25082146699634));
#13682=CARTESIAN_POINT('Ctrl Pts',(-0.125925468004263,6.63196518614269,
4.39924834947929));
#13683=CARTESIAN_POINT('Ctrl Pts',(-0.294649097744615,6.61762494437181,
4.42443992623928));
#13684=CARTESIAN_POINT('Ctrl Pts',(-0.439454924581737,6.60503562813921,
4.40266660815905));
#13685=CARTESIAN_POINT('Ctrl Pts',(-0.574832950582178,6.59240466995411,
4.33759318223502));
#13686=CARTESIAN_POINT('Ctrl Pts',(-0.696005607230916,6.57608629127481,
4.1858707309457));
#13687=CARTESIAN_POINT('Ctrl Pts',(-0.739264156798592,6.55968976182242,
3.99576554731973));
#13688=CARTESIAN_POINT('Ctrl Pts',(-0.688894544701315,6.54047191876598,
3.77281394895871));
#13689=CARTESIAN_POINT('Ctrl Pts',(-0.497850728795945,6.51838274700366,
3.58035881577739));
#13690=CARTESIAN_POINT('Ctrl Pts',(-0.226591456204558,6.49614979205781,
3.54992745923014));
#13691=CARTESIAN_POINT('Ctrl Pts',(-0.0170228957665506,6.47659384394549,
3.65124693095961));
#13692=CARTESIAN_POINT('Ctrl Pts',(0.107878534876526,6.45976489129137,3.80756740153316));
#13693=CARTESIAN_POINT('Ctrl Pts',(0.148935258357734,6.44427701128731,3.98728011631239));
#13694=CARTESIAN_POINT('Ctrl Pts',(0.121070920781021,6.43015138549249,4.15108396416147));
#13695=CARTESIAN_POINT('Ctrl Pts',(0.0485868461854486,6.41740335767032,
4.28244796483226));
#13696=CARTESIAN_POINT('Ctrl Pts',(-0.0635788152688685,6.40462128856916,
4.38248248865166));
#13697=CARTESIAN_POINT('Ctrl Pts',(-0.249190470547445,6.38753474317254,
4.45995182159303));
#13698=CARTESIAN_POINT('Ctrl Pts',(-0.510621805419283,6.36609553105664,
4.43099932549576));
#13699=CARTESIAN_POINT('Ctrl Pts',(-0.735220544630679,6.3402506864649,4.20663986268119));
#13700=CARTESIAN_POINT('Ctrl Pts',(-0.770998171812698,6.31429203879871,
3.89005168056026));
#13701=CARTESIAN_POINT('Ctrl Pts',(-0.601002821637636,6.28823331590632,
3.61892894068927));
#13702=CARTESIAN_POINT('Ctrl Pts',(-0.348588870206163,6.26643951526414,
3.53076923929659));
#13703=CARTESIAN_POINT('Ctrl Pts',(-0.145904386441107,6.24896558866351,
3.56564777464724));
#13704=CARTESIAN_POINT('Ctrl Pts',(0.00431784369931261,6.23438222817505,
3.64842497686876));
#13705=CARTESIAN_POINT('Ctrl Pts',(0.123537769777284,6.21831525558541,3.79782624277368));
#13706=CARTESIAN_POINT('Ctrl Pts',(0.170025222345384,6.20075900678011,4.0014515149975));
#13707=CARTESIAN_POINT('Ctrl Pts',(0.127382100777052,6.18464189141261,4.18835406447036));
#13708=CARTESIAN_POINT('Ctrl Pts',(0.0274168012845219,6.16997297685647,
4.32905626517445));
#13709=CARTESIAN_POINT('Ctrl Pts',(-0.0993153752368822,6.15675918917126,
4.41905554753229));
#13710=CARTESIAN_POINT('Ctrl Pts',(-0.248808689491018,6.14353471820731,
4.46210209715592));
#13711=CARTESIAN_POINT('Ctrl Pts',(-0.421546420510728,6.12883206416157,
4.45249609505736));
#13712=CARTESIAN_POINT('Ctrl Pts',(-0.594922024953856,6.11264861980656,
4.36896482777448));
#13713=CARTESIAN_POINT('Ctrl Pts',(-0.726050316003777,6.09498288711894,
4.20473974459702));
#13714=CARTESIAN_POINT('Ctrl Pts',(-0.772757113366257,6.07731254500321,
3.99981370250454));
#13715=CARTESIAN_POINT('Ctrl Pts',(-0.726037252404702,6.05963671350822,
3.79481962943994));
#13716=CARTESIAN_POINT('Ctrl Pts',(-0.594870280365665,6.04196116089001,
3.63048998551027));
#13717=CARTESIAN_POINT('Ctrl Pts',(-0.437085933471611,6.02723405694994,
3.55447714399662));
#13718=CARTESIAN_POINT('Ctrl Pts',(-0.300449841085889,6.01545653985552,
3.53917140938389));
#13719=CARTESIAN_POINT('Ctrl Pts',(-0.198020627129986,6.00662573148117,
3.55068011444686));
#13720=CARTESIAN_POINT('Ctrl Pts',(-0.10076495902483,5.99779697154375,3.58474829480414));
#13721=CARTESIAN_POINT('Ctrl Pts',(0.0156022323485835,5.98602915164187,
3.65776634877876));
#13722=CARTESIAN_POINT('Ctrl Pts',(0.124579597342358,5.97132617166562,3.79450200461182));
#13723=CARTESIAN_POINT('Ctrl Pts',(0.171307599715364,5.95369881069723,3.99892400350196));
#13724=CARTESIAN_POINT('Ctrl Pts',(0.124586125732732,5.93609064773941,4.20309708206352));
#13725=CARTESIAN_POINT('Ctrl Pts',(0.00506039749480362,5.91997078621416,
4.35300358200538));
#13726=CARTESIAN_POINT('Ctrl Pts',(-0.145693538275405,5.9053358357862,4.43620069859275));
#13727=CARTESIAN_POINT('Ctrl Pts',(-0.298307108656463,5.89217919980634,
4.46217466683996));
#13728=CARTESIAN_POINT('Ctrl Pts',(-0.4506139703325,5.87903967195749,4.43616034004319));
#13729=CARTESIAN_POINT('Ctrl Pts',(-0.631049677432172,5.86154513447298,
4.33689323122855));
#13730=CARTESIAN_POINT('Ctrl Pts',(-0.773616196183908,5.83972276022349,
4.11032978657596));
#13731=CARTESIAN_POINT('Ctrl Pts',(-0.737476573839881,5.81362592603361,
3.7917862723857));
#13732=CARTESIAN_POINT('Ctrl Pts',(-0.511745890186628,5.78762592348582,
3.5663291033827));
#13733=CARTESIAN_POINT('Ctrl Pts',(-0.195652728007556,5.76173371775045,
3.53089989430616));
#13734=CARTESIAN_POINT('Ctrl Pts',(0.0271465436298084,5.74025186815025,
3.67148645494915));
#13735=CARTESIAN_POINT('Ctrl Pts',(0.124242507955019,5.723131520039,3.84810446118424));
#13736=CARTESIAN_POINT('Ctrl Pts',(0.141141112031897,5.7145929194544,3.94698799978555));
#13737=CARTESIAN_POINT('Ctrl Pts',(0.141147803406803,5.71032999235489,3.99658474166685));
#13738=CARTESIAN_POINT('Ctrl Pts',(0.0442569588189985,7.0373337582885,3.99890379365327));
#13739=CARTESIAN_POINT('Ctrl Pts',(0.044251720623501,7.03399662424325,4.0377294577401));
#13740=CARTESIAN_POINT('Ctrl Pts',(0.0310421174065812,7.02733438487718,
4.11487645730137));
#13741=CARTESIAN_POINT('Ctrl Pts',(-0.044520373619987,7.0140191496109,4.25222378524957));
#13742=CARTESIAN_POINT('Ctrl Pts',(-0.217092875989633,6.9973934512664,4.36083736886208));
#13743=CARTESIAN_POINT('Ctrl Pts',(-0.460362141449961,6.97746421899541,
4.33337109400074));
#13744=CARTESIAN_POINT('Ctrl Pts',(-0.633229581407061,6.95754409339033,
4.16044956838266));
#13745=CARTESIAN_POINT('Ctrl Pts',(-0.660649519608787,6.93762277079198,
3.9173921089824));
#13746=CARTESIAN_POINT('Ctrl Pts',(-0.530497743214058,6.91768886249792,
3.71017764393557));
#13747=CARTESIAN_POINT('Ctrl Pts',(-0.299219066943147,6.89773161738857,
3.62914591381445));
#13748=CARTESIAN_POINT('Ctrl Pts',(-0.0762481443875615,6.8784802155694,
3.70724406195172));
#13749=CARTESIAN_POINT('Ctrl Pts',(0.0504447451103739,6.85993019956411,
3.89325360676551));
#13750=CARTESIAN_POINT('Ctrl Pts',(0.0507270478770132,6.8420804059587,4.1097457930552));
#13751=CARTESIAN_POINT('Ctrl Pts',(-0.061345173924128,6.82567116808314,
4.27427218667378));
#13752=CARTESIAN_POINT('Ctrl Pts',(-0.221824833436464,6.81071112770432,
4.35136044287204));
#13753=CARTESIAN_POINT('Ctrl Pts',(-0.382377722888624,6.79721237823048,
4.35143578641661));
#13754=CARTESIAN_POINT('Ctrl Pts',(-0.527460201032351,6.78367653739436,
4.2815814647059));
#13755=CARTESIAN_POINT('Ctrl Pts',(-0.628251688517972,6.77009810114687,
4.1553667808244));
#13756=CARTESIAN_POINT('Ctrl Pts',(-0.664300918515711,6.75647582308053,
3.99739333351463));
#13757=CARTESIAN_POINT('Ctrl Pts',(-0.628247832683737,6.74280717262616,
3.83886658894804));
#13758=CARTESIAN_POINT('Ctrl Pts',(-0.526580608007555,6.72908872568232,
3.71121541326947));
#13759=CARTESIAN_POINT('Ctrl Pts',(-0.379000812565982,6.71531747846208,
3.64009790518248));
#13760=CARTESIAN_POINT('Ctrl Pts',(-0.214574935364114,6.70149202624025,
3.64001889290798));
#13761=CARTESIAN_POINT('Ctrl Pts',(-0.0656866478755031,6.68760926695514,
3.71161277891696));
#13762=CARTESIAN_POINT('Ctrl Pts',(0.0376362054416423,6.6736673626485,3.84121263629532));
#13763=CARTESIAN_POINT('Ctrl Pts',(0.0792800261450241,6.65810712777825,
4.02168616321321));
#13764=CARTESIAN_POINT('Ctrl Pts',(0.0179396503705256,6.64090166096957,
4.22114376447229));
#13765=CARTESIAN_POINT('Ctrl Pts',(-0.146252315151375,6.62358638474026,
4.35224015227077));
#13766=CARTESIAN_POINT('Ctrl Pts',(-0.295254695663572,6.61092185793103,
4.37448789694979));
#13767=CARTESIAN_POINT('Ctrl Pts',(-0.423135906675798,6.59980383275673,
4.35525987816847));
#13768=CARTESIAN_POINT('Ctrl Pts',(-0.542699558880315,6.58864825053648,
4.29779214729782));
#13769=CARTESIAN_POINT('Ctrl Pts',(-0.649748287956536,6.5742326725394,4.16376617529517));
#13770=CARTESIAN_POINT('Ctrl Pts',(-0.687992729133971,6.55974144076396,
3.99575416152389));
#13771=CARTESIAN_POINT('Ctrl Pts',(-0.643465150667448,6.54274640684286,
3.79858751496941));
#13772=CARTESIAN_POINT('Ctrl Pts',(-0.474396005533634,6.52319303697642,
3.62818230613942));
#13773=CARTESIAN_POINT('Ctrl Pts',(-0.233899438524157,6.50348113431911,
3.60112665283043));
#13774=CARTESIAN_POINT('Ctrl Pts',(-0.0477706845000143,6.48611482218327,
3.69107139148393));
#13775=CARTESIAN_POINT('Ctrl Pts',(0.06333604123178,6.47114764580443,3.83007984654435));
#13776=CARTESIAN_POINT('Ctrl Pts',(0.099942513815026,6.45735180967165,3.99015866708828));
#13777=CARTESIAN_POINT('Ctrl Pts',(0.0750991629903671,6.44474937141879,
4.13630617444996));
#13778=CARTESIAN_POINT('Ctrl Pts',(0.0103545698946879,6.43336007312552,
4.25368042396433));
#13779=CARTESIAN_POINT('Ctrl Pts',(-0.0899993132508311,6.42192347736188,
4.34320250093748));
#13780=CARTESIAN_POINT('Ctrl Pts',(-0.256324344794604,6.40661143299051,
4.4126505577667));
#13781=CARTESIAN_POINT('Ctrl Pts',(-0.491200921321888,6.38735277795623,
4.3867749537966));
#13782=CARTESIAN_POINT('Ctrl Pts',(-0.693833157267625,6.36405139407747,
4.18461691050123));
#13783=CARTESIAN_POINT('Ctrl Pts',(-0.726414474840098,6.34056093669188,
3.89809595710794));
#13784=CARTESIAN_POINT('Ctrl Pts',(-0.57209606869426,6.31688067742868,3.65157253476251));
#13785=CARTESIAN_POINT('Ctrl Pts',(-0.34174487852591,6.2969914003347,3.57092118513008));
#13786=CARTESIAN_POINT('Ctrl Pts',(-0.156064544641843,6.28098618732206,
3.60283127144748));
#13787=CARTESIAN_POINT('Ctrl Pts',(-0.0181211835377871,6.26759749754076,
3.67880681109718));
#13788=CARTESIAN_POINT('Ctrl Pts',(0.0917071518592229,6.25280461900015,
3.81633040921865));
#13789=CARTESIAN_POINT('Ctrl Pts',(0.134725986725988,6.23658646287139,4.0044321517635));
#13790=CARTESIAN_POINT('Ctrl Pts',(0.0952665525924826,6.2216474183188,4.17770434573801));
#13791=CARTESIAN_POINT('Ctrl Pts',(0.00234826205902896,6.20800987537027,
4.30855288182894));
#13792=CARTESIAN_POINT('Ctrl Pts',(-0.115777655276309,6.19569304278798,
4.39248379346406));
#13793=CARTESIAN_POINT('Ctrl Pts',(-0.255507423162007,6.18333388843454,
4.43275482656015));
#13794=CARTESIAN_POINT('Ctrl Pts',(-0.417424148324254,6.1695541663508,4.42379163882968));
#13795=CARTESIAN_POINT('Ctrl Pts',(-0.580494199072148,6.15433738090676,
4.34530507136999));
#13796=CARTESIAN_POINT('Ctrl Pts',(-0.704336977323806,6.13766622912363,
4.19035189958122));
#13797=CARTESIAN_POINT('Ctrl Pts',(-0.748674915963105,6.12092336607669,
3.99618742403465));
#13798=CARTESIAN_POINT('Ctrl Pts',(-0.704328759622937,6.10411386533969,
3.80118099794721));
#13799=CARTESIAN_POINT('Ctrl Pts',(-0.579138032632301,6.08723770701643,
3.64420072065554));
#13800=CARTESIAN_POINT('Ctrl Pts',(-0.427899020685579,6.07312085586337,
3.57125725585403));
#13801=CARTESIAN_POINT('Ctrl Pts',(-0.296498016849044,6.06179556804166,
3.55652395581677));
#13802=CARTESIAN_POINT('Ctrl Pts',(-0.197792520819203,6.05328612269475,
3.56760248202455));
#13803=CARTESIAN_POINT('Ctrl Pts',(-0.103880776642972,6.04476202684289,
3.60048749552585));
#13804=CARTESIAN_POINT('Ctrl Pts',(0.00871742473144576,6.03337695875632,
3.67111939944296));
#13805=CARTESIAN_POINT('Ctrl Pts',(0.114534197432594,6.01911078308422,3.80376795494684));
#13806=CARTESIAN_POINT('Ctrl Pts',(0.160165391665353,6.00193635608825,4.00294447276823));
#13807=CARTESIAN_POINT('Ctrl Pts',(0.114532721808726,5.98470952374257,4.20275174445739));
#13808=CARTESIAN_POINT('Ctrl Pts',(-0.00284531791589128,5.9688722885223,
4.3501044912035));
#13809=CARTESIAN_POINT('Ctrl Pts',(-0.151509186623747,5.9544396588332,4.43219617802463));
#13810=CARTESIAN_POINT('Ctrl Pts',(-0.302485556876914,5.94142572331473,
4.45793192009972));
#13811=CARTESIAN_POINT('Ctrl Pts',(-0.453653070305428,5.92838747414629,
4.43214963221505));
#13812=CARTESIAN_POINT('Ctrl Pts',(-0.633313395400228,5.91097204664598,
4.33337553358166));
#13813=CARTESIAN_POINT('Ctrl Pts',(-0.776152268672977,5.88915102619383,
4.10690588901937));
#13814=CARTESIAN_POINT('Ctrl Pts',(-0.740125674897743,5.86288681368008,
3.78621135475587));
#13815=CARTESIAN_POINT('Ctrl Pts',(-0.511714727939696,5.8365560405257,3.55759037145094));
#13816=CARTESIAN_POINT('Ctrl Pts',(-0.189550345441767,5.81016809980556,
3.52112644113214));
#13817=CARTESIAN_POINT('Ctrl Pts',(0.0391040166061708,5.78814007529024,
3.66511438089066));
#13818=CARTESIAN_POINT('Ctrl Pts',(0.139214121292207,5.77049985171582,3.84708655092079));
#13819=CARTESIAN_POINT('Ctrl Pts',(0.156700985320598,5.76167201173322,3.9493235059236));
#13820=CARTESIAN_POINT('Ctrl Pts',(0.156707905565383,5.75726327669175,4.00061664061033));
#13821=CARTESIAN_POINT('Ctrl Pts',(0.0751457037399773,6.99854476807283,
3.99557397917139));
#13822=CARTESIAN_POINT('Ctrl Pts',(0.075140007219866,6.99491564594273,4.03779675921048));
#13823=CARTESIAN_POINT('Ctrl Pts',(0.0607581710523704,6.98766756923154,
4.1217301725566));
#13824=CARTESIAN_POINT('Ctrl Pts',(-0.0212194890442437,6.97323144469361,
4.27063232486073));
#13825=CARTESIAN_POINT('Ctrl Pts',(-0.207586513843011,6.9552906871778,4.38769413865131));
#13826=CARTESIAN_POINT('Ctrl Pts',(-0.468424025791189,6.93392328513651,
4.35794023955));
#13827=CARTESIAN_POINT('Ctrl Pts',(-0.652319413050973,6.91271075698153,
4.17355011831035));
#13828=CARTESIAN_POINT('Ctrl Pts',(-0.680999823764982,6.89164674870683,
3.91645876707414));
#13829=CARTESIAN_POINT('Ctrl Pts',(-0.544080453606905,6.87072405599895,
3.69908687220202));
#13830=CARTESIAN_POINT('Ctrl Pts',(-0.3029915213572,6.84993503879299,3.61497227631154));
#13831=CARTESIAN_POINT('Ctrl Pts',(-0.0725787408381743,6.83003719070295,
3.69601298637691));
#13832=CARTESIAN_POINT('Ctrl Pts',(0.0572211404977879,6.81100671844234,
3.88702167820545));
#13833=CARTESIAN_POINT('Ctrl Pts',(0.0572773755168048,6.79282253208309,
4.10760648245781));
#13834=CARTESIAN_POINT('Ctrl Pts',(-0.0562661565167663,6.77622751890747,
4.27390914776326));
#13835=CARTESIAN_POINT('Ctrl Pts',(-0.217603410728839,6.76119500558845,
4.35128302310882));
#13836=CARTESIAN_POINT('Ctrl Pts',(-0.378103579756139,6.74770325553529,
4.3512621445762));
#13837=CARTESIAN_POINT('Ctrl Pts',(-0.522312778460912,6.73424518629264,
4.28171670475117));
#13838=CARTESIAN_POINT('Ctrl Pts',(-0.621904906869197,6.72082120908127,
4.15685139905434));
#13839=CARTESIAN_POINT('Ctrl Pts',(-0.657262086760371,6.70742610962714,
4.00146518682517));
#13840=CARTESIAN_POINT('Ctrl Pts',(-0.621901886731202,6.69405663540931,
3.84640605158284));
#13841=CARTESIAN_POINT('Ctrl Pts',(-0.522899910822995,6.6807105640045,3.72225590441482));
#13842=CARTESIAN_POINT('Ctrl Pts',(-0.380021303489903,6.66738551430775,
3.65350850640738));
#13843=CARTESIAN_POINT('Ctrl Pts',(-0.221699556245957,6.65407642679375,
3.6535238424819));
#13844=CARTESIAN_POINT('Ctrl Pts',(-0.0791142190191431,6.64078122645618,
3.72219044199103));
#13845=CARTESIAN_POINT('Ctrl Pts',(0.0192972475475469,6.62749562655119,
3.8457679781254));
#13846=CARTESIAN_POINT('Ctrl Pts',(0.0586956163165313,6.61274299064652,
4.01696310984453));
#13847=CARTESIAN_POINT('Ctrl Pts',(0.00066375925222291,6.59651620933359,
4.2050275731726));
#13848=CARTESIAN_POINT('Ctrl Pts',(-0.153334584529499,6.58029099014053,
4.32775376427335));
#13849=CARTESIAN_POINT('Ctrl Pts',(-0.292259119428385,6.5684849763937,4.34842537504501));
#13850=CARTESIAN_POINT('Ctrl Pts',(-0.411147701512788,6.55814961736179,
4.33054329311896));
#13851=CARTESIAN_POINT('Ctrl Pts',(-0.521955614976932,6.54781050041763,
4.27721853387123));
#13852=CARTESIAN_POINT('Ctrl Pts',(-0.620725061677617,6.53450259960706,
4.15344094423789));
#13853=CARTESIAN_POINT('Ctrl Pts',(-0.65582099214931,6.52118134802923,3.9989509292853));
#13854=CARTESIAN_POINT('Ctrl Pts',(-0.61495699708586,6.50561562040471,3.81836101275701));
#13855=CARTESIAN_POINT('Ctrl Pts',(-0.460662252093786,6.4877934967267,3.66313033402));
#13856=CARTESIAN_POINT('Ctrl Pts',(-0.242482824178419,6.46991415829505,
3.63876953283619));
#13857=CARTESIAN_POINT('Ctrl Pts',(-0.0743337604068055,6.45422487028971,
3.7201015694052));
#13858=CARTESIAN_POINT('Ctrl Pts',(0.0257354859861971,6.44073974504913,
3.84538128706963));
#13859=CARTESIAN_POINT('Ctrl Pts',(0.0585804358516633,6.4283462329255,3.9892205820693));
#13860=CARTESIAN_POINT('Ctrl Pts',(0.0362872215500701,6.4170485024808,4.1202410123795));
#13861=CARTESIAN_POINT('Ctrl Pts',(-0.0216702917476953,6.40685673434529,
4.22527201055116));
#13862=CARTESIAN_POINT('Ctrl Pts',(-0.111335998722885,6.39664004540801,
4.30523794358292));
#13863=CARTESIAN_POINT('Ctrl Pts',(-0.259711447124339,6.38298245740987,
4.36716519030964));
#13864=CARTESIAN_POINT('Ctrl Pts',(-0.46875010272031,6.36584361765854,4.34403783761716));
#13865=CARTESIAN_POINT('Ctrl Pts',(-0.648586756900391,6.34515613291672,
4.16448041223341));
#13866=CARTESIAN_POINT('Ctrl Pts',(-0.677373174728768,6.32434544881345,
3.91060268518533));
#13867=CARTESIAN_POINT('Ctrl Pts',(-0.540800891160044,6.30339796777644,
3.69254462095115));
#13868=CARTESIAN_POINT('Ctrl Pts',(-0.337234792203235,6.28582440056116,
3.62130867843882));
#13869=CARTESIAN_POINT('Ctrl Pts',(-0.173237146150972,6.27168848386102,
3.64949647834371));
#13870=CARTESIAN_POINT('Ctrl Pts',(-0.051430185488775,6.2598663781925,3.71658825071815));
#13871=CARTESIAN_POINT('Ctrl Pts',(0.04553624276142,6.24680590347271,3.83800936553293));
#13872=CARTESIAN_POINT('Ctrl Pts',(0.0835203927235832,6.23248666293686,
4.00408895192877));
#13873=CARTESIAN_POINT('Ctrl Pts',(0.0486781044779186,6.21929378875258,
4.15710891455627));
#13874=CARTESIAN_POINT('Ctrl Pts',(-0.0334048064306245,6.20724619112471,
4.27270501202057));
#13875=CARTESIAN_POINT('Ctrl Pts',(-0.137798620671507,6.19636086286606,
4.34688345273625));
#13876=CARTESIAN_POINT('Ctrl Pts',(-0.261348178132289,6.18543268369284,
4.38249551422101));
#13877=CARTESIAN_POINT('Ctrl Pts',(-0.404602265285608,6.17324102985752,
4.37457199336662));
#13878=CARTESIAN_POINT('Ctrl Pts',(-0.549002049255003,6.15976710926115,
4.30508999673435));
#13879=CARTESIAN_POINT('Ctrl Pts',(-0.658795353214431,6.14498870842845,
4.16774772662554));
#13880=CARTESIAN_POINT('Ctrl Pts',(-0.698173399037309,6.13012858235954,
3.99542272969115));
#13881=CARTESIAN_POINT('Ctrl Pts',(-0.658783439304685,6.11518723031923,
3.82209155039728));
#13882=CARTESIAN_POINT('Ctrl Pts',(-0.547360330742578,6.10016316209671,
3.68232226746707));
#13883=CARTESIAN_POINT('Ctrl Pts',(-0.412501870305111,6.0875735567346,3.61724796858836));
#13884=CARTESIAN_POINT('Ctrl Pts',(-0.295158341169763,6.07745968950951,
3.60408403079106));
#13885=CARTESIAN_POINT('Ctrl Pts',(-0.20692700197197,6.0698531511466,3.61398247465688));
#13886=CARTESIAN_POINT('Ctrl Pts',(-0.122893280869518,6.06222564151618,
3.64340341424773));
#13887=CARTESIAN_POINT('Ctrl Pts',(-0.0220334947688963,6.05202741453606,
3.70666465199554));
#13888=CARTESIAN_POINT('Ctrl Pts',(0.0729349027491596,6.03922702577368,
3.82565491225774));
#13889=CARTESIAN_POINT('Ctrl Pts',(0.114014005851098,6.02378160903268,4.00475544378273));
#13890=CARTESIAN_POINT('Ctrl Pts',(0.0729309939381365,6.00825150319719,
4.18488477257113));
#13891=CARTESIAN_POINT('Ctrl Pts',(-0.0331103150260445,5.99393771535338,
4.31808397533113));
#13892=CARTESIAN_POINT('Ctrl Pts',(-0.167763499397065,5.98086359359795,
4.39247080088669));
#13893=CARTESIAN_POINT('Ctrl Pts',(-0.304804591381143,5.9690494019362,4.41585679085843));
#13894=CARTESIAN_POINT('Ctrl Pts',(-0.442321747056314,5.95718795428887,
4.39242706556015));
#13895=CARTESIAN_POINT('Ctrl Pts',(-0.606120129125199,5.94131003833698,
4.30241537837807));
#13896=CARTESIAN_POINT('Ctrl Pts',(-0.736935222086037,5.92134505674546,
4.09535276040965));
#13897=CARTESIAN_POINT('Ctrl Pts',(-0.704063817046733,5.897202863713,3.8005784837169));
#13898=CARTESIAN_POINT('Ctrl Pts',(-0.493262956617019,5.87287814300756,
3.58923924816358));
#13899=CARTESIAN_POINT('Ctrl Pts',(-0.194189503439066,5.84837693048783,
3.55511225114028));
#13900=CARTESIAN_POINT('Ctrl Pts',(0.0193738527175865,5.82781135703401,
3.68933048543546));
#13901=CARTESIAN_POINT('Ctrl Pts',(0.113245033351325,5.81127961886183,3.85984437961461));
#13902=CARTESIAN_POINT('Ctrl Pts',(0.129703151080226,5.80298162751628,3.95593314931651));
#13903=CARTESIAN_POINT('Ctrl Pts',(0.129709662131318,5.79883358073614,4.00419332376098));
#13904=CARTESIAN_POINT('Ctrl Pts',(0.124798013448484,6.99868851973232,3.99559303376014));
#13905=CARTESIAN_POINT('Ctrl Pts',(0.124791575197003,6.99458685758227,4.04331354923134));
#13906=CARTESIAN_POINT('Ctrl Pts',(0.108519340653653,6.98638331383568,4.13830928780707));
#13907=CARTESIAN_POINT('Ctrl Pts',(0.0157294368859061,6.97004260916147,
4.30685622612404));
#13908=CARTESIAN_POINT('Ctrl Pts',(-0.195313267658951,6.94972310181207,
4.43944484961639));
#13909=CARTESIAN_POINT('Ctrl Pts',(-0.490725500432085,6.92552221004534,
4.4057409716263));
#13910=CARTESIAN_POINT('Ctrl Pts',(-0.698906971683536,6.90150379307887,
4.19696215792743));
#13911=CARTESIAN_POINT('Ctrl Pts',(-0.731302466905495,6.87767190209846,
3.90610635189342));
#13912=CARTESIAN_POINT('Ctrl Pts',(-0.57652734771189,6.85402790905394,3.66052645769687));
#13913=CARTESIAN_POINT('Ctrl Pts',(-0.304524133193118,6.83057351697921,
3.56572939296188));
#13914=CARTESIAN_POINT('Ctrl Pts',(-0.0451810802227447,6.80817096763108,
3.65706578636171));
#13915=CARTESIAN_POINT('Ctrl Pts',(0.10050224257138,6.78679665612694,3.87162772975011));
#13916=CARTESIAN_POINT('Ctrl Pts',(0.100457763025169,6.76642768238877,4.11869777142394));
#13917=CARTESIAN_POINT('Ctrl Pts',(-0.0264325451155999,6.74789297827438,
4.30435282479636));
#13918=CARTESIAN_POINT('Ctrl Pts',(-0.206109828879609,6.7311512513616,4.39045119843915));
#13919=CARTESIAN_POINT('Ctrl Pts',(-0.384343980705665,6.71616672905262,
4.39036989044689));
#13920=CARTESIAN_POINT('Ctrl Pts',(-0.543993429740019,6.70126503100192,
4.31331397713504));
#13921=CARTESIAN_POINT('Ctrl Pts',(-0.65388167053252,6.68644371689127,4.1754321737649));
#13922=CARTESIAN_POINT('Ctrl Pts',(-0.692721455623035,6.67170290736964,
4.00444785555966));
#13923=CARTESIAN_POINT('Ctrl Pts',(-0.653879336914907,6.6570414842913,3.83444051025451));
#13924=CARTESIAN_POINT('Ctrl Pts',(-0.545657981513214,6.64245786103533,
3.69884639844091));
#13925=CARTESIAN_POINT('Ctrl Pts',(-0.390109756917324,6.62795015317063,
3.62408934269625));
#13926=CARTESIAN_POINT('Ctrl Pts',(-0.218468583985697,6.61351806688075,
3.62418508472824));
#13927=CARTESIAN_POINT('Ctrl Pts',(-0.0645595410678361,6.59915930397135,
3.69840045898558));
#13928=CARTESIAN_POINT('Ctrl Pts',(0.0411765748371212,6.58487294660812,
3.83130376244869));
#13929=CARTESIAN_POINT('Ctrl Pts',(0.083247757435789,6.56907615945228,4.01458173082189));
#13930=CARTESIAN_POINT('Ctrl Pts',(0.0212844204770885,6.55180018803028,
4.2147383509278));
#13931=CARTESIAN_POINT('Ctrl Pts',(-0.141775654108723,6.53462919748218,
4.34442182713541));
#13932=CARTESIAN_POINT('Ctrl Pts',(-0.287926289336259,6.52220689767782,
4.36608503842369));
#13933=CARTESIAN_POINT('Ctrl Pts',(-0.412575975619086,6.51136947179089,
4.34732797703399));
#13934=CARTESIAN_POINT('Ctrl Pts',(-0.528343188394878,6.5005621516852,4.29153814826038));
#13935=CARTESIAN_POINT('Ctrl Pts',(-0.630947515877118,6.48672638390543,
4.16279511909207));
#13936=CARTESIAN_POINT('Ctrl Pts',(-0.667156630704825,6.47294344017427,
4.00298851862108));
#13937=CARTESIAN_POINT('Ctrl Pts',(-0.624997276978197,6.45692653478884,
3.81720227944088));
#13938=CARTESIAN_POINT('Ctrl Pts',(-0.467057927631317,6.4387005619605,3.65873827571917));
#13939=CARTESIAN_POINT('Ctrl Pts',(-0.245834304281332,6.4205698163312,3.63434388139158));
#13940=CARTESIAN_POINT('Ctrl Pts',(-0.0765730344102318,6.40476511714423,
3.71634854532427));
#13941=CARTESIAN_POINT('Ctrl Pts',(0.0235696507731436,6.39125997399593,
3.84186810089354));
#13942=CARTESIAN_POINT('Ctrl Pts',(0.0561947006325922,6.3789107097248,3.98516908431952));
#13943=CARTESIAN_POINT('Ctrl Pts',(0.0340532508098388,6.36770980799088,
4.11504089990853));
#13944=CARTESIAN_POINT('Ctrl Pts',(-0.0232053258500781,6.35764612467795,
4.21871751604287));
#13945=CARTESIAN_POINT('Ctrl Pts',(-0.111393660303079,6.34759820362209,
4.29731940679757));
#13946=CARTESIAN_POINT('Ctrl Pts',(-0.256738526493721,6.33422090775404,
4.35791879870519));
#13947=CARTESIAN_POINT('Ctrl Pts',(-0.460216792556107,6.31753050026247,
4.33514023261262));
#13948=CARTESIAN_POINT('Ctrl Pts',(-0.633672374499552,6.29754795827952,
4.16149374392549));
#13949=CARTESIAN_POINT('Ctrl Pts',(-0.660949637255133,6.27759198565784,
3.91813756683918));
#13950=CARTESIAN_POINT('Ctrl Pts',(-0.53077931166136,6.25765964857123,3.71087969162022));
#13951=CARTESIAN_POINT('Ctrl Pts',(-0.33846821757528,6.24105542601477,3.64383802463471));
#13952=CARTESIAN_POINT('Ctrl Pts',(-0.184444074251402,6.22777510682923,
3.67036091043645));
#13953=CARTESIAN_POINT('Ctrl Pts',(-0.0704339054081569,6.2167058919551,
3.7331989943449));
#13954=CARTESIAN_POINT('Ctrl Pts',(0.0199204368139329,6.20452621499493,
3.84646102936634));
#13955=CARTESIAN_POINT('Ctrl Pts',(0.0551098304872991,6.19123118680399,
4.00065923711283));
#13956=CARTESIAN_POINT('Ctrl Pts',(0.0228302131702101,6.1790331648205,4.14210729423421));
#13957=CARTESIAN_POINT('Ctrl Pts',(-0.0528133398235512,6.16793255456529,
4.24857750065134));
#13958=CARTESIAN_POINT('Ctrl Pts',(-0.148722501496592,6.15793189937884,
4.31668991376579));
#13959=CARTESIAN_POINT('Ctrl Pts',(-0.261896992548591,6.14791939152312,
4.34928384757038));
#13960=CARTESIAN_POINT('Ctrl Pts',(-0.392743709961473,6.13678179173137,
4.34201524293595));
#13961=CARTESIAN_POINT('Ctrl Pts',(-0.524209299176861,6.1245107719564,4.27870091640551));
#13962=CARTESIAN_POINT('Ctrl Pts',(-0.623804592783382,6.11109541704753,
4.1540163818384));
#13963=CARTESIAN_POINT('Ctrl Pts',(-0.659377157185489,6.09765172267441,
3.99811930846562));
#13964=CARTESIAN_POINT('Ctrl Pts',(-0.62379462303483,6.08417214571078,3.8417901780194));
#13965=CARTESIAN_POINT('Ctrl Pts',(-0.523543767573635,6.07065633465871,
3.71610462448052));
#13966=CARTESIAN_POINT('Ctrl Pts',(-0.402545085275045,6.05936021527247,
3.6577583409882));
#13967=CARTESIAN_POINT('Ctrl Pts',(-0.297471872035578,6.0503031208645,3.6459761452668));
#13968=CARTESIAN_POINT('Ctrl Pts',(-0.218558620392158,6.04349971284653,
3.65483446064));
#13969=CARTESIAN_POINT('Ctrl Pts',(-0.143482710344404,6.03668462484246,
3.68112357015323));
#13970=CARTESIAN_POINT('Ctrl Pts',(-0.0534709391286362,6.02758246181735,
3.73758932459396));
#13971=CARTESIAN_POINT('Ctrl Pts',(0.0311419308736091,6.01617355264696,
3.8436466619805));
#13972=CARTESIAN_POINT('Ctrl Pts',(0.0676526336744417,6.00243252914066,
4.00297467696501));
#13973=CARTESIAN_POINT('Ctrl Pts',(0.0311452431252221,5.98863818021461,
4.16294558794561));
#13974=CARTESIAN_POINT('Ctrl Pts',(-0.0629151833074351,5.97594279894951,
4.28106220629714));
#13975=CARTESIAN_POINT('Ctrl Pts',(-0.182207296201302,5.9643598495178,4.34695436925805));
#13976=CARTESIAN_POINT('Ctrl Pts',(-0.303519296564873,5.95390085955684,
4.36765003397419));
#13977=CARTESIAN_POINT('Ctrl Pts',(-0.425166618854115,5.94340734969263,
4.34691962242895));
#13978=CARTESIAN_POINT('Ctrl Pts',(-0.569977269229313,5.92936902647442,
4.26733379692996));
#13979=CARTESIAN_POINT('Ctrl Pts',(-0.685535786419193,5.91172770302844,
4.08438020509818));
#13980=CARTESIAN_POINT('Ctrl Pts',(-0.656499898140925,5.89040718152557,
3.82407675111926));
#13981=CARTESIAN_POINT('Ctrl Pts',(-0.470369297569495,5.86892675166902,
3.63744932630136));
#13982=CARTESIAN_POINT('Ctrl Pts',(-0.206193885052881,5.84728307371841,
3.60727155581054));
#13983=CARTESIAN_POINT('Ctrl Pts',(-0.0173782093166548,5.82910240014456,
3.72587589968568));
#13984=CARTESIAN_POINT('Ctrl Pts',(0.0656915399010325,5.81447418238888,
3.87675001240063));
#13985=CARTESIAN_POINT('Ctrl Pts',(0.0802681551442859,5.80712809467601,
3.9618129389144));
#13986=CARTESIAN_POINT('Ctrl Pts',(0.0802739273614817,5.8034507426456,4.00459684659137));
#13987=CARTESIAN_POINT('Ctrl Pts',(0.155898286953838,7.03728022619773,3.99891425465501));
#13988=CARTESIAN_POINT('Ctrl Pts',(0.155891381493523,7.03288091602972,4.0500977361937));
#13989=CARTESIAN_POINT('Ctrl Pts',(0.138432195279057,7.02407113276436,4.15211258318849));
#13990=CARTESIAN_POINT('Ctrl Pts',(0.038565797916663,7.00647506231035,4.33361879406262));
#13991=CARTESIAN_POINT('Ctrl Pts',(-0.189473518840625,6.9845044451475,4.47714449100908));
#13992=CARTESIAN_POINT('Ctrl Pts',(-0.510457801790799,6.95820850684306,
4.4408079840861));
#13993=CARTESIAN_POINT('Ctrl Pts',(-0.737915267426515,6.93198498747228,
4.21308019321558));
#13994=CARTESIAN_POINT('Ctrl Pts',(-0.773692800313957,6.90584663337165,
3.89414328734837));
#13995=CARTESIAN_POINT('Ctrl Pts',(-0.603422771103904,6.87980181841352,
3.62353526879945));
#13996=CARTESIAN_POINT('Ctrl Pts',(-0.302681629986891,6.85386056759999,
3.51849097457158));
#13997=CARTESIAN_POINT('Ctrl Pts',(-0.0147058400958794,6.8289880657698,
3.6197102775808));
#13998=CARTESIAN_POINT('Ctrl Pts',(0.147679051850326,6.80517848086569,3.85863003203219));
#13999=CARTESIAN_POINT('Ctrl Pts',(0.147745220775547,6.78242389077341,4.1346283406934));
#14000=CARTESIAN_POINT('Ctrl Pts',(0.00570064244535932,6.76166320926415,
4.34263115496595));
#14001=CARTESIAN_POINT('Ctrl Pts',(-0.195956608936766,6.74287152561178,
4.43931546269542));
#14002=CARTESIAN_POINT('Ctrl Pts',(-0.396340311853144,6.72602487978657,
4.43926157585714));
#14003=CARTESIAN_POINT('Ctrl Pts',(-0.576112450455779,6.70924619472044,
4.35252925292814));
#14004=CARTESIAN_POINT('Ctrl Pts',(-0.700030850777678,6.69253636270515,
4.19709322386811));
#14005=CARTESIAN_POINT('Ctrl Pts',(-0.74389769318666,6.67589771458627,4.00409528410642));
#14006=CARTESIAN_POINT('Ctrl Pts',(-0.700031510087649,6.65933220722945,
3.81199668730109));
#14007=CARTESIAN_POINT('Ctrl Pts',(-0.577663754631793,6.64284110408447,
3.65864746207902));
#14008=CARTESIAN_POINT('Ctrl Pts',(-0.401654106030834,6.62642604558861,
3.5740381158214));
#14009=CARTESIAN_POINT('Ctrl Pts',(-0.207333431610751,6.61008845759303,
3.57413426225354));
#14010=CARTESIAN_POINT('Ctrl Pts',(-0.0330325771222907,6.59382967848166,
3.65817267563611));
#14011=CARTESIAN_POINT('Ctrl Pts',(0.0867249114115746,6.57765070813198,
3.8086949886927));
#14012=CARTESIAN_POINT('Ctrl Pts',(0.134373312114564,6.55976435473091,4.01625437067971));
#14013=CARTESIAN_POINT('Ctrl Pts',(0.064200943600672,6.54020522159148,4.24286346201966));
#14014=CARTESIAN_POINT('Ctrl Pts',(-0.12029152798752,6.52078200916156,4.38955907374434));
#14015=CARTESIAN_POINT('Ctrl Pts',(-0.285487765251715,6.50674266719864,
4.41402855850721));
#14016=CARTESIAN_POINT('Ctrl Pts',(-0.426292318861567,6.49450160484564,
4.39284001400122));
#14017=CARTESIAN_POINT('Ctrl Pts',(-0.55695886060963,6.48230474083829,4.32985048339294));
#14018=CARTESIAN_POINT('Ctrl Pts',(-0.672616264480391,6.4667067066286,4.1846858955765));
#14019=CARTESIAN_POINT('Ctrl Pts',(-0.713347999015104,6.45119483968567,
4.00478575277996));
#14020=CARTESIAN_POINT('Ctrl Pts',(-0.66592845882305,6.43319552875216,3.79598496681771));
#14021=CARTESIAN_POINT('Ctrl Pts',(-0.4887581341486,6.4127691710153,3.6183946156295));
#14022=CARTESIAN_POINT('Ctrl Pts',(-0.241498728326516,6.39250941732578,
3.59127281368563));
#14023=CARTESIAN_POINT('Ctrl Pts',(-0.0529425060409864,6.37490536021007,
3.68269376647733));
#14024=CARTESIAN_POINT('Ctrl Pts',(0.0583085954390705,6.35989710487152,
3.82222366005482));
#14025=CARTESIAN_POINT('Ctrl Pts',(0.0944075756390824,6.34621737094437,
3.98102240423213));
#14026=CARTESIAN_POINT('Ctrl Pts',(0.0699085235340198,6.33383941511541,
4.12455298430901));
#14027=CARTESIAN_POINT('Ctrl Pts',(0.00675161232934667,6.32274498294321,
4.23885320140307));
#14028=CARTESIAN_POINT('Ctrl Pts',(-0.090256633454611,6.31169591385856,
4.32527973589332));
#14029=CARTESIAN_POINT('Ctrl Pts',(-0.249726812385787,6.29702309261973,
4.39172521686747));
#14030=CARTESIAN_POINT('Ctrl Pts',(-0.472018088461371,6.27879476792815,
4.36662957913525));
#14031=CARTESIAN_POINT('Ctrl Pts',(-0.660259735570777,6.25708995257749,
4.17779412869095));
#14032=CARTESIAN_POINT('Ctrl Pts',(-0.689429979510665,6.23555833236324,
3.91502853353564));
#14033=CARTESIAN_POINT('Ctrl Pts',(-0.549544978189975,6.21418573888641,
3.69285774823168));
#14034=CARTESIAN_POINT('Ctrl Pts',(-0.344583867661803,6.1965076698517,3.62166594025428));
#14035=CARTESIAN_POINT('Ctrl Pts',(-0.181357894942747,6.1824356292938,3.64982599888188));
#14036=CARTESIAN_POINT('Ctrl Pts',(-0.0609759353177233,6.17074988836366,
3.71622172910107));
#14037=CARTESIAN_POINT('Ctrl Pts',(0.0339738702340465,6.15794530953578,
3.83537372624937));
#14038=CARTESIAN_POINT('Ctrl Pts',(0.070699027192326,6.14403681879006,3.99673460654441));
#14039=CARTESIAN_POINT('Ctrl Pts',(0.0370178729943884,6.13134114386906,
4.14396432017652));
#14040=CARTESIAN_POINT('Ctrl Pts',(-0.0414034061013744,6.11984114333799,
4.25426713362554));
#14041=CARTESIAN_POINT('Ctrl Pts',(-0.140420083399158,6.10952207378331,
4.32454338637078));
#14042=CARTESIAN_POINT('Ctrl Pts',(-0.256779120536252,6.09923333420609,
4.35801270993916));
#14043=CARTESIAN_POINT('Ctrl Pts',(-0.390772964435132,6.08783113368769,
4.3505251901726));
#14044=CARTESIAN_POINT('Ctrl Pts',(-0.524724794165585,6.0753273372258,4.28590847874342));
#14045=CARTESIAN_POINT('Ctrl Pts',(-0.625616062768487,6.06173420831728,
4.15945493331342));
#14046=CARTESIAN_POINT('Ctrl Pts',(-0.661381460593111,6.04818027154711,
4.00223728641184));
#14047=CARTESIAN_POINT('Ctrl Pts',(-0.625613714016865,6.03466962836758,
3.84550094762344));
#14048=CARTESIAN_POINT('Ctrl Pts',(-0.525551501680262,6.0211951913812,3.72022382017239));
#14049=CARTESIAN_POINT('Ctrl Pts',(-0.405502332613917,6.00999486905733,
3.66242421459593));
#14050=CARTESIAN_POINT('Ctrl Pts',(-0.301695807990352,6.00104844401153,
3.65080398560401));
#14051=CARTESIAN_POINT('Ctrl Pts',(-0.223942524395158,5.99434541683584,
3.65954297266594));
#14052=CARTESIAN_POINT('Ctrl Pts',(-0.150177426985106,5.98764995088656,
3.68538608217118));
#14053=CARTESIAN_POINT('Ctrl Pts',(-0.0619734954203226,5.97873123536758,
3.74073401474671));
#14054=CARTESIAN_POINT('Ctrl Pts',(0.0205383989162633,5.96760036580935,
3.84428791195509));
#14055=CARTESIAN_POINT('Ctrl Pts',(0.0558943829569689,5.95426466640533,
3.99898167490483));
#14056=CARTESIAN_POINT('Ctrl Pts',(0.0205364233023731,5.94094754169309,
4.15343929607048));
#14057=CARTESIAN_POINT('Ctrl Pts',(-0.0698977870616078,5.92875347004186,
4.26686649595146));
#14058=CARTESIAN_POINT('Ctrl Pts',(-0.184027799874841,5.91767538066872,
4.32985348664582));
#14059=CARTESIAN_POINT('Ctrl Pts',(-0.299632781229378,5.90771186407747,
4.34953322344785));
#14060=CARTESIAN_POINT('Ctrl Pts',(-0.415115100018854,5.89775216087867,
4.32981503807356));
#14061=CARTESIAN_POINT('Ctrl Pts',(-0.552081340816604,5.88447527420849,
4.25447792316758));
#14062=CARTESIAN_POINT('Ctrl Pts',(-0.660599511459815,5.86788715437798,
4.08221655549765));
#14063=CARTESIAN_POINT('Ctrl Pts',(-0.633187418646854,5.84797211597177,
3.83902623944222));
#14064=CARTESIAN_POINT('Ctrl Pts',(-0.460232598593138,5.82804167779231,
3.66597042270737));
#14065=CARTESIAN_POINT('Ctrl Pts',(-0.21651953940244,5.80808128197822,3.63839308255855));
#14066=CARTESIAN_POINT('Ctrl Pts',(-0.0435016794216495,5.79141903729581,
3.74729104993654));
#14067=CARTESIAN_POINT('Ctrl Pts',(0.0323279853604166,5.77805814895842,
3.88511820484604));
#14068=CARTESIAN_POINT('Ctrl Pts',(0.0455846737864788,5.77137052102706,
3.96257235116211));
#14069=CARTESIAN_POINT('Ctrl Pts',(0.0455899333128428,5.76801979299628,
4.00155617363396));
#14070=CARTESIAN_POINT('Ctrl Pts',(0.144678245631215,7.08554680213199,4.00306133790045));
#14071=CARTESIAN_POINT('Ctrl Pts',(0.144671500355495,7.08124954188956,4.05305752636765));
#14072=CARTESIAN_POINT('Ctrl Pts',(0.127638295897203,7.07264307654079,4.15273372378903));
#14073=CARTESIAN_POINT('Ctrl Pts',(0.0297906758184221,7.05539141371109,
4.33071621748334));
#14074=CARTESIAN_POINT('Ctrl Pts',(-0.194624694461135,7.03376092249549,
4.47227310994897));
#14075=CARTESIAN_POINT('Ctrl Pts',(-0.512793689617035,7.0077016180938,4.43660565671338));
#14076=CARTESIAN_POINT('Ctrl Pts',(-0.739891117513686,6.98155185240586,
4.20969228951669));
#14077=CARTESIAN_POINT('Ctrl Pts',(-0.776134874518362,6.95532017556054,
3.88959979024378));
#14078=CARTESIAN_POINT('Ctrl Pts',(-0.604430469514607,6.92901725042124,
3.61607628645324));
#14079=CARTESIAN_POINT('Ctrl Pts',(-0.298850270112994,6.90265311426136,
3.5089773670217));
#14080=CARTESIAN_POINT('Ctrl Pts',(-0.0041877729162317,6.87721684305035,
3.6122029034201));
#14081=CARTESIAN_POINT('Ctrl Pts',(0.163085243952079,6.8527238294967,3.85787769361227));
#14082=CARTESIAN_POINT('Ctrl Pts',(0.163384882825869,6.82918609064528,4.14338542492333));
#14083=CARTESIAN_POINT('Ctrl Pts',(0.015823003083378,6.80759518268656,4.35983941897781));
#14084=CARTESIAN_POINT('Ctrl Pts',(-0.19485297859053,6.78796098573423,4.46096458777198));
#14085=CARTESIAN_POINT('Ctrl Pts',(-0.405068526852833,6.77028845501068,
4.46099811143608));
#14086=CARTESIAN_POINT('Ctrl Pts',(-0.594442506826705,6.75261759300039,
4.36973390477035));
#14087=CARTESIAN_POINT('Ctrl Pts',(-0.725521830010195,6.73495168097432,
4.20545805379156));
#14088=CARTESIAN_POINT('Ctrl Pts',(-0.772159744972474,6.7172940852679,4.00065424379591));
#14089=CARTESIAN_POINT('Ctrl Pts',(-0.725515499865608,6.69964790652088,
3.79600816012752));
#14090=CARTESIAN_POINT('Ctrl Pts',(-0.594752448164995,6.68201643280477,
3.63200459373353));
#14091=CARTESIAN_POINT('Ctrl Pts',(-0.405927741373564,6.66440258324841,
3.54114672713638));
#14092=CARTESIAN_POINT('Ctrl Pts',(-0.196685934801451,6.64680993881577,
3.5411729761552));
#14093=CARTESIAN_POINT('Ctrl Pts',(-0.00831861674380411,6.62924133491153,
3.63190747468183));
#14094=CARTESIAN_POINT('Ctrl Pts',(0.121572695078818,6.61170024961743,3.79505321054773));
#14095=CARTESIAN_POINT('Ctrl Pts',(0.173479639665487,6.59224330272307,4.02079117854625));
#14096=CARTESIAN_POINT('Ctrl Pts',(0.0970225484155485,6.57088994378068,
4.26823368838363));
#14097=CARTESIAN_POINT('Ctrl Pts',(-0.105126136635525,6.54959621783657,
4.42916044832145));
#14098=CARTESIAN_POINT('Ctrl Pts',(-0.286826829701903,6.53415291663596,
4.4561321994847));
#14099=CARTESIAN_POINT('Ctrl Pts',(-0.441985250736035,6.52066326933656,
4.43278777827631));
#14100=CARTESIAN_POINT('Ctrl Pts',(-0.586261220893134,6.50719630370112,
4.36328940520075));
#14101=CARTESIAN_POINT('Ctrl Pts',(-0.714326528660687,6.48993058540335,
4.20264640858163));
#14102=CARTESIAN_POINT('Ctrl Pts',(-0.759578088890916,6.47271357412861,
4.00301451687559));
#14103=CARTESIAN_POINT('Ctrl Pts',(-0.706890145842292,6.4526901815544,3.77074626745266));
#14104=CARTESIAN_POINT('Ctrl Pts',(-0.509348264358454,6.42989539310044,
3.57253036910641));
#14105=CARTESIAN_POINT('Ctrl Pts',(-0.232673374234872,6.4072213283679,3.54204681697485));
#14106=CARTESIAN_POINT('Ctrl Pts',(-0.0211606489794148,6.38747158289537,
3.64454937174464));
#14107=CARTESIAN_POINT('Ctrl Pts',(0.10385050553,6.37061025692699,3.80127847521638));
#14108=CARTESIAN_POINT('Ctrl Pts',(0.144499767686605,6.35521294411437,3.97996599015471));
#14109=CARTESIAN_POINT('Ctrl Pts',(0.11691297736442,6.34126688370014,4.14166635350243));
#14110=CARTESIAN_POINT('Ctrl Pts',(0.0457037622501119,6.32875467680033,
4.2705620245579));
#14111=CARTESIAN_POINT('Ctrl Pts',(-0.0637765139051123,6.31628241125697,
4.36811362660792));
#14112=CARTESIAN_POINT('Ctrl Pts',(-0.243887986166721,6.29970752541662,
4.44317377591863));
#14113=CARTESIAN_POINT('Ctrl Pts',(-0.495229957712618,6.27909069195944,
4.41484962337697));
#14114=CARTESIAN_POINT('Ctrl Pts',(-0.708286432087431,6.25452486128724,
4.20117890011158));
#14115=CARTESIAN_POINT('Ctrl Pts',(-0.741330918581209,6.23012937021185,
3.90363242728255));
#14116=CARTESIAN_POINT('Ctrl Pts',(-0.582907516210337,6.2059161665878,3.65203300687903));
#14117=CARTESIAN_POINT('Ctrl Pts',(-0.350842144541872,6.18588854891781,
3.57145512299382));
#14118=CARTESIAN_POINT('Ctrl Pts',(-0.16616267347381,6.16996303930852,3.60332715230888));
#14119=CARTESIAN_POINT('Ctrl Pts',(-0.0300193261453657,6.1567431579809,
3.6784240642902));
#14120=CARTESIAN_POINT('Ctrl Pts',(0.0772697082943915,6.14226898651452,
3.81309635659369));
#14121=CARTESIAN_POINT('Ctrl Pts',(0.118711944999288,6.1265634666449,3.99528114055935));
#14122=CARTESIAN_POINT('Ctrl Pts',(0.0806988497789685,6.11224384637075,
4.16130380343939));
#14123=CARTESIAN_POINT('Ctrl Pts',(-0.00764523437737332,6.09928702591431,
4.2855359239597));
#14124=CARTESIAN_POINT('Ctrl Pts',(-0.119061347128016,6.08767307012448,
4.36458894128047));
#14125=CARTESIAN_POINT('Ctrl Pts',(-0.249824643571864,6.07610587445443,
4.40218494533652));
#14126=CARTESIAN_POINT('Ctrl Pts',(-0.400178064050431,6.06330773686186,
4.39376127834984));
#14127=CARTESIAN_POINT('Ctrl Pts',(-0.550214494811022,6.04929754952555,
4.32135094499318));
#14128=CARTESIAN_POINT('Ctrl Pts',(-0.662945002779939,6.03409632303652,
4.1799671043587));
#14129=CARTESIAN_POINT('Ctrl Pts',(-0.702782576913764,6.01898178761487,
4.00466261722736));
#14130=CARTESIAN_POINT('Ctrl Pts',(-0.662935573975121,6.00394761901098,
3.83034152873934));
#14131=CARTESIAN_POINT('Ctrl Pts',(-0.551913042299725,5.98899659078265,
3.69142024206081));
#14132=CARTESIAN_POINT('Ctrl Pts',(-0.419127185826005,5.97660551336272,
3.62754451453377));
#14133=CARTESIAN_POINT('Ctrl Pts',(-0.304612679823387,5.96673442572674,
3.61473293745679));
#14134=CARTESIAN_POINT('Ctrl Pts',(-0.218980861908636,5.95935166909097,
3.62436627546611));
#14135=CARTESIAN_POINT('Ctrl Pts',(-0.137875282342012,5.95198838173858,
3.65278906578636));
#14136=CARTESIAN_POINT('Ctrl Pts',(-0.0410640067172789,5.94219726798964,
3.71355547533596));
#14137=CARTESIAN_POINT('Ctrl Pts',(0.0492362339959224,5.93000589656047,
3.82697125746778));
#14138=CARTESIAN_POINT('Ctrl Pts',(0.0877277228792333,5.91545396739186,
3.99574063387158));
#14139=CARTESIAN_POINT('Ctrl Pts',(0.0492465765145144,5.90097796291407,
4.16356675179509));
#14140=CARTESIAN_POINT('Ctrl Pts',(-0.0486820579380837,5.88777724801351,
4.28628146889304));
#14141=CARTESIAN_POINT('Ctrl Pts',(-0.171751854364245,5.87583082210482,
4.35416544596331));
#14142=CARTESIAN_POINT('Ctrl Pts',(-0.296013425129878,5.86511834632131,
4.37528682708976));
#14143=CARTESIAN_POINT('Ctrl Pts',(-0.419716281141755,5.85444563424213,
4.35413476774134));
#14144=CARTESIAN_POINT('Ctrl Pts',(-0.565929655577575,5.84026767787951,
4.27365549771028));
#14145=CARTESIAN_POINT('Ctrl Pts',(-0.680990719323017,5.8226369137051,4.09054212894091));
#14146=CARTESIAN_POINT('Ctrl Pts',(-0.651757681535579,5.80162737226418,
3.83412076912136));
#14147=CARTESIAN_POINT('Ctrl Pts',(-0.470477481012713,5.78075525660051,
3.65319906029932));
#14148=CARTESIAN_POINT('Ctrl Pts',(-0.217264499890463,5.76001348508868,
3.62489033715765));
#14149=CARTESIAN_POINT('Ctrl Pts',(-0.0390539840425255,5.74283038603375,
3.7373503101674));
#14150=CARTESIAN_POINT('Ctrl Pts',(0.0385809790069335,5.72913985701358,
3.87858381898698));
#14151=CARTESIAN_POINT('Ctrl Pts',(0.0520898426589243,5.722316450254,3.95760322649394));
#14152=CARTESIAN_POINT('Ctrl Pts',(0.0520952028928984,5.71890156362907,
3.99733349786329));
#14153=CARTESIAN_POINT('Ctrl Pts',(0.1149593871984,7.09981632447119,4.00428381887363));
#14154=CARTESIAN_POINT('Ctrl Pts',(0.114953085439515,7.0958016186183,4.05099264708923));
#14155=CARTESIAN_POINT('Ctrl Pts',(0.0990499949612588,7.08776451642407,
4.1440749819009));
#14156=CARTESIAN_POINT('Ctrl Pts',(0.00756609025685691,7.07163054708052,
4.3105312207836));
#14157=CARTESIAN_POINT('Ctrl Pts',(-0.20265191966924,7.05136317960048,4.4432442233264));
#14158=CARTESIAN_POINT('Ctrl Pts',(-0.501576002622839,7.02688068565122,
4.40988522403664));
#14159=CARTESIAN_POINT('Ctrl Pts',(-0.715649296673727,7.00224333371635,
4.19621127354387));
#14160=CARTESIAN_POINT('Ctrl Pts',(-0.750065379754911,6.977454834481,3.89375410180805));
#14161=CARTESIAN_POINT('Ctrl Pts',(-0.587448639243598,6.95252105745876,
3.63437652438941));
#14162=CARTESIAN_POINT('Ctrl Pts',(-0.296883906961772,6.92744748855256,
3.53234593196161));
#14163=CARTESIAN_POINT('Ctrl Pts',(-0.0156214196491875,6.90317435214424,
3.63068646565069));
#14164=CARTESIAN_POINT('Ctrl Pts',(0.144662679260828,6.87972358982664,3.86584230232094));
#14165=CARTESIAN_POINT('Ctrl Pts',(0.145088543148844,6.85711434464457,4.14009778924436));
#14166=CARTESIAN_POINT('Ctrl Pts',(0.00298259309759907,6.83630747956724,
4.3487833250613));
#14167=CARTESIAN_POINT('Ctrl Pts',(-0.200629153718379,6.8173312082382,4.44659816529074));
#14168=CARTESIAN_POINT('Ctrl Pts',(-0.404350038818084,6.80020649499647,
4.44669337921948));
#14169=CARTESIAN_POINT('Ctrl Pts',(-0.588383432588771,6.78303663281808,
4.35806872308743));
#14170=CARTESIAN_POINT('Ctrl Pts',(-0.716130694480413,6.76582937646054,
4.19807595671414));
#14171=CARTESIAN_POINT('Ctrl Pts',(-0.76174697024645,6.74858383891329,3.99803802216038));
#14172=CARTESIAN_POINT('Ctrl Pts',(-0.716126250508271,6.7313025559897,3.79758613790949));
#14173=CARTESIAN_POINT('Ctrl Pts',(-0.58775583974693,6.71398953196761,3.63647816172447));
#14174=CARTESIAN_POINT('Ctrl Pts',(-0.401838339917565,6.69664899601872,
3.54694262619554));
#14175=CARTESIAN_POINT('Ctrl Pts',(-0.195214549156962,6.67928042967714,
3.54690060253338));
#14176=CARTESIAN_POINT('Ctrl Pts',(-0.00865722368073337,6.66188873083374,
3.63668289231812));
#14177=CARTESIAN_POINT('Ctrl Pts',(0.120374244388054,6.64447474921385,3.79864518662284));
#14178=CARTESIAN_POINT('Ctrl Pts',(0.172141661215916,6.62510839439489,4.02339166080862));
#14179=CARTESIAN_POINT('Ctrl Pts',(0.095889564871484,6.60377546807264,4.27065330650525));
#14180=CARTESIAN_POINT('Ctrl Pts',(-0.106719746155468,6.58242925442276,
4.4321448062933));
#14181=CARTESIAN_POINT('Ctrl Pts',(-0.289520583900008,6.5668956717895,4.45933997294184));
#14182=CARTESIAN_POINT('Ctrl Pts',(-0.445921222784358,6.55329978788634,
4.4358156174397));
#14183=CARTESIAN_POINT('Ctrl Pts',(-0.591635462985678,6.53970440462415,
4.36567953699744));
#14184=CARTESIAN_POINT('Ctrl Pts',(-0.721389666696936,6.52221950596346,
4.20303067518927));
#14185=CARTESIAN_POINT('Ctrl Pts',(-0.767405188483471,6.50474251981698,
4.000316390915));
#14186=CARTESIAN_POINT('Ctrl Pts',(-0.713830810800694,6.48435445670912,
3.76376923070465));
#14187=CARTESIAN_POINT('Ctrl Pts',(-0.51214130973696,6.46107773227755,3.56109836625548));
#14188=CARTESIAN_POINT('Ctrl Pts',(-0.228267597822158,6.43781873998792,
3.5296222132148));
#14189=CARTESIAN_POINT('Ctrl Pts',(-0.0104681813815427,6.41749488904288,
3.63508347114042));
#14190=CARTESIAN_POINT('Ctrl Pts',(0.118638327797451,6.40008799366429,3.79685627397656));
#14191=CARTESIAN_POINT('Ctrl Pts',(0.160770132095208,6.38415833960461,3.98178426841228));
#14192=CARTESIAN_POINT('Ctrl Pts',(0.132174615335124,6.36969190973263,4.14955144088928));
#14193=CARTESIAN_POINT('Ctrl Pts',(0.0581767737661934,6.35668810557578,
4.2835498059508));
#14194=CARTESIAN_POINT('Ctrl Pts',(-0.0558338873469698,6.34370163075499,
4.38516402527543));
#14195=CARTESIAN_POINT('Ctrl Pts',(-0.243754538377708,6.32640951048581,
4.46351775255043));
#14196=CARTESIAN_POINT('Ctrl Pts',(-0.506762819769542,6.30484691807606,
4.43403489872079));
#14197=CARTESIAN_POINT('Ctrl Pts',(-0.730668971919691,6.27905054023632,
4.20975403365834));
#14198=CARTESIAN_POINT('Ctrl Pts',(-0.765678686873786,6.25335957707319,
3.89618560227291));
#14199=CARTESIAN_POINT('Ctrl Pts',(-0.59828824591992,6.22776564997827,3.63001002509955));
#14200=CARTESIAN_POINT('Ctrl Pts',(-0.35211960915011,6.20653414885713,3.54438589454075));
#14201=CARTESIAN_POINT('Ctrl Pts',(-0.155684959604055,6.18960076014007,
3.57825744186559));
#14202=CARTESIAN_POINT('Ctrl Pts',(-0.010661377238107,6.1755244002249,3.65822950437421));
#14203=CARTESIAN_POINT('Ctrl Pts',(0.103859085093381,6.1600835663691,3.80190427731936));
#14204=CARTESIAN_POINT('Ctrl Pts',(0.148204575463535,6.14329585710035,3.99667156211874));
#14205=CARTESIAN_POINT('Ctrl Pts',(0.107533874360454,6.12796192084666,4.17450217859232));
#14206=CARTESIAN_POINT('Ctrl Pts',(0.0127852845025076,6.11406789381457,
4.3077723562051));
#14207=CARTESIAN_POINT('Ctrl Pts',(-0.106861005480655,6.1015991481364,4.39269001253556));
#14208=CARTESIAN_POINT('Ctrl Pts',(-0.247456764966195,6.0891678153038,4.43312715503312));
#14209=CARTESIAN_POINT('Ctrl Pts',(-0.409327203073403,6.07539362335861,
4.42407672254863));
#14210=CARTESIAN_POINT('Ctrl Pts',(-0.571069625287454,6.06029537121561,
4.34603758409293));
#14211=CARTESIAN_POINT('Ctrl Pts',(-0.692783271109274,6.04389453255034,
4.19344865326311));
#14212=CARTESIAN_POINT('Ctrl Pts',(-0.735861926194011,6.0275588239698,4.00395604220365));
#14213=CARTESIAN_POINT('Ctrl Pts',(-0.692776967423399,6.01129753338503,
3.81531844116176));
#14214=CARTESIAN_POINT('Ctrl Pts',(-0.572513817468236,5.99510729772473,
3.6648179318568));
#14215=CARTESIAN_POINT('Ctrl Pts',(-0.428536498276722,5.98167596786366,
3.5955416477389));
#14216=CARTESIAN_POINT('Ctrl Pts',(-0.304268279887566,5.97096604692344,
3.58164029219959));
#14217=CARTESIAN_POINT('Ctrl Pts',(-0.211302708259727,5.96295150211699,
3.59209575299587));
#14218=CARTESIAN_POINT('Ctrl Pts',(-0.123221561998884,5.95495625976633,
3.62296222963301));
#14219=CARTESIAN_POINT('Ctrl Pts',(-0.0180442464683113,5.9443206556865,
3.68897371165251));
#14220=CARTESIAN_POINT('Ctrl Pts',(0.0800964737981796,5.93107533649748,
3.81222858617156));
#14221=CARTESIAN_POINT('Ctrl Pts',(0.121963800542189,5.91525638154566,3.99573810944841));
#14222=CARTESIAN_POINT('Ctrl Pts',(0.0800951474414264,5.89951422438799,
4.17829694994921));
#14223=CARTESIAN_POINT('Ctrl Pts',(-0.0264610976803377,5.88515352693233,
4.31182517350449));
#14224=CARTESIAN_POINT('Ctrl Pts',(-0.160404840361885,5.87215362307701,
4.38570130500428));
#14225=CARTESIAN_POINT('Ctrl Pts',(-0.295639561854143,5.86049817284501,
4.40868318905617));
#14226=CARTESIAN_POINT('Ctrl Pts',(-0.430262394364154,5.8488860820304,4.38565877817388));
#14227=CARTESIAN_POINT('Ctrl Pts',(-0.589366688691013,5.83346068619404,
4.29807824715954));
#14228=CARTESIAN_POINT('Ctrl Pts',(-0.714505317186666,5.81429088075568,
4.09887385317267));
#14229=CARTESIAN_POINT('Ctrl Pts',(-0.68268303776338,5.79145791366774,3.82012733243894));
#14230=CARTESIAN_POINT('Ctrl Pts',(-0.485773655554561,5.7687981740651,3.62368921351975));
#14231=CARTESIAN_POINT('Ctrl Pts',(-0.211134005665917,5.74630660226991,
3.59306391087273));
#14232=CARTESIAN_POINT('Ctrl Pts',(-0.0182181343487706,5.72770693474824,
3.71490466632272));
#14233=CARTESIAN_POINT('Ctrl Pts',(0.0657101590335888,5.71290424256539,
3.86762790031566));
#14234=CARTESIAN_POINT('Ctrl Pts',(0.0802918585875821,5.70553413368605,
3.95299047765578));
#14235=CARTESIAN_POINT('Ctrl Pts',(0.0802976428954483,5.7018490789545,3.99586400189706));
#14236=CARTESIAN_POINT('Ctrl Pts',(0.0999994223174587,7.09981632447119,
4.00428180053801));
#14237=CARTESIAN_POINT('Ctrl Pts',(0.0999933436797077,7.09594376396835,
4.04933684813297));
#14238=CARTESIAN_POINT('Ctrl Pts',(0.0846594327171957,7.08819408394972,
4.13908992957458));
#14239=CARTESIAN_POINT('Ctrl Pts',(-0.00357043069494361,7.07263318914228,
4.29963340285418));
#14240=CARTESIAN_POINT('Ctrl Pts',(-0.206356294917572,7.05308143195573,
4.42766373470968));
#14241=CARTESIAN_POINT('Ctrl Pts',(-0.494863120131574,7.02945164505109,
4.39548903188326));
#14242=CARTESIAN_POINT('Ctrl Pts',(-0.701612481834811,7.00565862484048,
4.18915927264886));
#14243=CARTESIAN_POINT('Ctrl Pts',(-0.734902354617378,6.98170298771966,
3.89687986754614));
#14244=CARTESIAN_POINT('Ctrl Pts',(-0.577665286755769,6.9575878275568,3.64601239877861));
#14245=CARTESIAN_POINT('Ctrl Pts',(-0.296425446296891,6.93331589731144,
3.54721069783272));
#14246=CARTESIAN_POINT('Ctrl Pts',(-0.0238970429973844,6.90979548741706,
3.64245102870328));
#14247=CARTESIAN_POINT('Ctrl Pts',(0.131586191166419,6.88704931445005,3.8704985271515));
#14248=CARTESIAN_POINT('Ctrl Pts',(0.132036205657411,6.86509836852865,4.13674945418924));
#14249=CARTESIAN_POINT('Ctrl Pts',(-0.0060413687179679,6.84487478558125,
4.33958298894643));
#14250=CARTESIAN_POINT('Ctrl Pts',(-0.204116844890033,6.82641141958407,
4.43475944317313));
#14251=CARTESIAN_POINT('Ctrl Pts',(-0.402473369433673,6.80973569344043,
4.43486896119673));
#14252=CARTESIAN_POINT('Ctrl Pts',(-0.581827228221285,6.79300305116116,
4.34852221416367));
#14253=CARTESIAN_POINT('Ctrl Pts',(-0.706454134874152,6.7762153628094,4.192464816352));
#14254=CARTESIAN_POINT('Ctrl Pts',(-0.751016294559626,6.75937457420164,
3.99715087739011));
#14255=CARTESIAN_POINT('Ctrl Pts',(-0.706447662037028,6.74248271608976,
3.80123388795173));
#14256=CARTESIAN_POINT('Ctrl Pts',(-0.580873534358325,6.72554188917784,
3.64359934962882));
#14257=CARTESIAN_POINT('Ctrl Pts',(-0.398793807750649,6.70855427056295,
3.55588854173989));
#14258=CARTESIAN_POINT('Ctrl Pts',(-0.196213186746174,6.69152210478501,
3.55582569363604));
#14259=CARTESIAN_POINT('Ctrl Pts',(-0.0130963934752721,6.67444770586136,
3.64392728654252));
#14260=CARTESIAN_POINT('Ctrl Pts',(0.113707820363769,6.65733344528682,3.80305624025719));
#14261=CARTESIAN_POINT('Ctrl Pts',(0.164656362590817,6.63827601697293,4.02413741573514));
#14262=CARTESIAN_POINT('Ctrl Pts',(0.0896082709820025,6.61726302509207,
4.2676978223342));
#14263=CARTESIAN_POINT('Ctrl Pts',(-0.110245732077343,6.59619863179822,
4.4270642600818));
#14264=CARTESIAN_POINT('Ctrl Pts',(-0.290838098938005,6.58084997747224,
4.45395573001046));
#14265=CARTESIAN_POINT('Ctrl Pts',(-0.445467117475853,6.56740673782488,
4.43069910759464));
#14266=CARTESIAN_POINT('Ctrl Pts',(-0.589663880409842,6.55395079532829,
4.36131796304211));
#14267=CARTESIAN_POINT('Ctrl Pts',(-0.718225707768932,6.53662851071928,
4.20020661739991));
#14268=CARTESIAN_POINT('Ctrl Pts',(-0.763898158866166,6.51928717897976,
3.99912848715837));
#14269=CARTESIAN_POINT('Ctrl Pts',(-0.710721419612997,6.49903664059857,
3.764202830041));
#14270=CARTESIAN_POINT('Ctrl Pts',(-0.510149997687367,6.47587070043553,
3.56253207697483));
#14271=CARTESIAN_POINT('Ctrl Pts',(-0.227250362890276,6.45268625633124,
3.53107252428385));
#14272=CARTESIAN_POINT('Ctrl Pts',(-0.00982453983942397,6.43239259089565,
3.63631313688574));
#14273=CARTESIAN_POINT('Ctrl Pts',(0.119224416062016,6.414995879623,3.79796488057796));
#14274=CARTESIAN_POINT('Ctrl Pts',(0.161414220224748,6.39904954972701,3.98302626625864));
#14275=CARTESIAN_POINT('Ctrl Pts',(0.132781651753175,6.38455548538367,4.15109736344141));
#14276=CARTESIAN_POINT('Ctrl Pts',(0.058591217696994,6.37151403493753,4.28547086198332));
#14277=CARTESIAN_POINT('Ctrl Pts',(-0.0558362639783319,6.35847699034469,
4.38747481451575));
#14278=CARTESIAN_POINT('Ctrl Pts',(-0.244624220570673,6.34110173177432,
4.46620946091905));
#14279=CARTESIAN_POINT('Ctrl Pts',(-0.509258386493358,6.31939963958705,
4.43663450707748));
#14280=CARTESIAN_POINT('Ctrl Pts',(-0.735030443095589,6.29339375292805,
4.21063569075453));
#14281=CARTESIAN_POINT('Ctrl Pts',(-0.770492148406669,6.2674338232997,3.89395438143295));
#14282=CARTESIAN_POINT('Ctrl Pts',(-0.601210048531917,6.24152902186401,
3.62457992816658));
#14283=CARTESIAN_POINT('Ctrl Pts',(-0.351688619951789,6.21999512440529,
3.53770552245775));
#14284=CARTESIAN_POINT('Ctrl Pts',(-0.152299417857812,6.20280445728418,
3.57207084012085));
#14285=CARTESIAN_POINT('Ctrl Pts',(-0.00495835013055459,6.18850033974624,
3.65330634586973));
#14286=CARTESIAN_POINT('Ctrl Pts',(0.111522803781729,6.17279483671223,3.79940640678234));
#14287=CARTESIAN_POINT('Ctrl Pts',(0.156701474788417,6.15570021231953,3.99770463755195));
#14288=CARTESIAN_POINT('Ctrl Pts',(0.115262604711903,6.14006777305336,4.17897821875209));
#14289=CARTESIAN_POINT('Ctrl Pts',(0.0185932180471106,6.12588811043834,
4.31497113433199));
#14290=CARTESIAN_POINT('Ctrl Pts',(-0.103590553659916,6.11315178814851,
4.4016989608744));
#14291=CARTESIAN_POINT('Ctrl Pts',(-0.247293954733903,6.1004417858412,4.44304193852122));
#14292=CARTESIAN_POINT('Ctrl Pts',(-0.412869049658234,6.08634982725544,
4.43379507168706));
#14293=CARTESIAN_POINT('Ctrl Pts',(-0.578482300908516,6.07088880084204,
4.3539190346138));
#14294=CARTESIAN_POINT('Ctrl Pts',(-0.703246723757797,6.05407432044984,
4.19753682982269));
#14295=CARTESIAN_POINT('Ctrl Pts',(-0.747469580607062,6.03731392465469,
4.00314057125818));
#14296=CARTESIAN_POINT('Ctrl Pts',(-0.703238625925696,6.02060951959296,
3.80940575329504));
#14297=CARTESIAN_POINT('Ctrl Pts',(-0.579634776479789,6.00396293095479,
3.65467865258803));
#14298=CARTESIAN_POINT('Ctrl Pts',(-0.431500759601328,5.99014040360805,
3.58338254073736));
#14299=CARTESIAN_POINT('Ctrl Pts',(-0.303561319206374,5.97911298339926,
3.56906449106088));
#14300=CARTESIAN_POINT('Ctrl Pts',(-0.207808748835976,5.97085791464426,
3.57983145987356));
#14301=CARTESIAN_POINT('Ctrl Pts',(-0.117044922248722,5.96261853714979,
3.6116348383249));
#14302=CARTESIAN_POINT('Ctrl Pts',(-0.00861997369778145,5.95165386736835,
3.67968231581426));
#14303=CARTESIAN_POINT('Ctrl Pts',(0.0926329081004657,5.93798817658918,
3.80681756846826));
#14304=CARTESIAN_POINT('Ctrl Pts',(0.135870644163702,5.92165495155963,3.99626375633351));
#14305=CARTESIAN_POINT('Ctrl Pts',(0.0926387969430078,5.90538860209907,
4.18487776410349));
#14306=CARTESIAN_POINT('Ctrl Pts',(-0.0175125738479973,5.89054016294629,
4.32293582509909));
#14307=CARTESIAN_POINT('Ctrl Pts',(-0.156061008534171,5.87709197920747,
4.39936287338782));
#14308=CARTESIAN_POINT('Ctrl Pts',(-0.296018497756522,5.86502791432804,
4.42315611503599));
#14309=CARTESIAN_POINT('Ctrl Pts',(-0.435406476921251,5.8530035361086,4.39932451423293));
#14310=CARTESIAN_POINT('Ctrl Pts',(-0.600212844195293,5.83702437044493,
4.30861645270809));
#14311=CARTESIAN_POINT('Ctrl Pts',(-0.729945333339283,5.81715142573852,
4.10216892170714));
#14312=CARTESIAN_POINT('Ctrl Pts',(-0.696976009348358,5.7934671926544,3.81306008549607));
#14313=CARTESIAN_POINT('Ctrl Pts',(-0.492652698548329,5.76994854996481,
3.60918617550531));
#14314=CARTESIAN_POINT('Ctrl Pts',(-0.207515825799976,5.74659510021081,
3.57736699868709));
#14315=CARTESIAN_POINT('Ctrl Pts',(-0.00714719245692835,5.72727465695078,
3.70390131122158));
#14316=CARTESIAN_POINT('Ctrl Pts',(0.0800330609517386,5.71189866882786,
3.86253474741929));
#14317=CARTESIAN_POINT('Ctrl Pts',(0.0951821641861108,5.70424160396714,
3.95121652410011));
#14318=CARTESIAN_POINT('Ctrl Pts',(0.0951881709252366,5.70041484319491,
3.99573871784903));
#14319=CARTESIAN_POINT('',(0.0999994223174587,7.09981632447119,4.00428180053802));
#14320=CARTESIAN_POINT('Origin',(0.1,7.05,4.));
#14321=CARTESIAN_POINT('',(0.0951881709252366,5.70041484319491,3.99573871784901));
#14322=CARTESIAN_POINT('Ctrl Pts',(0.0999994223174587,7.09981632447119,
4.00428180053801));
#14323=CARTESIAN_POINT('Ctrl Pts',(0.0999933436797077,7.09594376396835,
4.04933684813297));
#14324=CARTESIAN_POINT('Ctrl Pts',(0.0846594327171957,7.08819408394972,
4.13908992957458));
#14325=CARTESIAN_POINT('Ctrl Pts',(-0.00357043069494361,7.07263318914228,
4.29963340285418));
#14326=CARTESIAN_POINT('Ctrl Pts',(-0.206356294917572,7.05308143195573,
4.42766373470968));
#14327=CARTESIAN_POINT('Ctrl Pts',(-0.494863120131574,7.02945164505109,
4.39548903188326));
#14328=CARTESIAN_POINT('Ctrl Pts',(-0.701612481834811,7.00565862484048,
4.18915927264886));
#14329=CARTESIAN_POINT('Ctrl Pts',(-0.734902354617378,6.98170298771966,
3.89687986754614));
#14330=CARTESIAN_POINT('Ctrl Pts',(-0.577665286755769,6.9575878275568,3.64601239877861));
#14331=CARTESIAN_POINT('Ctrl Pts',(-0.296425446296891,6.93331589731144,
3.54721069783272));
#14332=CARTESIAN_POINT('Ctrl Pts',(-0.0238970429973844,6.90979548741706,
3.64245102870328));
#14333=CARTESIAN_POINT('Ctrl Pts',(0.131586191166419,6.88704931445005,3.8704985271515));
#14334=CARTESIAN_POINT('Ctrl Pts',(0.132036205657411,6.86509836852865,4.13674945418924));
#14335=CARTESIAN_POINT('Ctrl Pts',(-0.0060413687179679,6.84487478558125,
4.33958298894643));
#14336=CARTESIAN_POINT('Ctrl Pts',(-0.204116844890033,6.82641141958407,
4.43475944317313));
#14337=CARTESIAN_POINT('Ctrl Pts',(-0.402473369433673,6.80973569344043,
4.43486896119673));
#14338=CARTESIAN_POINT('Ctrl Pts',(-0.581827228221285,6.79300305116116,
4.34852221416367));
#14339=CARTESIAN_POINT('Ctrl Pts',(-0.706454134874152,6.7762153628094,4.192464816352));
#14340=CARTESIAN_POINT('Ctrl Pts',(-0.751016294559626,6.75937457420164,
3.99715087739011));
#14341=CARTESIAN_POINT('Ctrl Pts',(-0.706447662037028,6.74248271608976,
3.80123388795173));
#14342=CARTESIAN_POINT('Ctrl Pts',(-0.580873534358325,6.72554188917784,
3.64359934962882));
#14343=CARTESIAN_POINT('Ctrl Pts',(-0.398793807750649,6.70855427056295,
3.55588854173989));
#14344=CARTESIAN_POINT('Ctrl Pts',(-0.196213186746174,6.69152210478501,
3.55582569363604));
#14345=CARTESIAN_POINT('Ctrl Pts',(-0.0130963934752721,6.67444770586136,
3.64392728654252));
#14346=CARTESIAN_POINT('Ctrl Pts',(0.113707820363769,6.65733344528682,3.80305624025719));
#14347=CARTESIAN_POINT('Ctrl Pts',(0.164656362590817,6.63827601697293,4.02413741573514));
#14348=CARTESIAN_POINT('Ctrl Pts',(0.0896082709820025,6.61726302509207,
4.2676978223342));
#14349=CARTESIAN_POINT('Ctrl Pts',(-0.110245732077343,6.59619863179822,
4.4270642600818));
#14350=CARTESIAN_POINT('Ctrl Pts',(-0.290838098938005,6.58084997747224,
4.45395573001046));
#14351=CARTESIAN_POINT('Ctrl Pts',(-0.445467117475853,6.56740673782488,
4.43069910759464));
#14352=CARTESIAN_POINT('Ctrl Pts',(-0.589663880409842,6.55395079532829,
4.36131796304211));
#14353=CARTESIAN_POINT('Ctrl Pts',(-0.718225707768932,6.53662851071928,
4.20020661739991));
#14354=CARTESIAN_POINT('Ctrl Pts',(-0.763898158866166,6.51928717897976,
3.99912848715837));
#14355=CARTESIAN_POINT('Ctrl Pts',(-0.710721419612997,6.49903664059857,
3.764202830041));
#14356=CARTESIAN_POINT('Ctrl Pts',(-0.510149997687367,6.47587070043553,
3.56253207697483));
#14357=CARTESIAN_POINT('Ctrl Pts',(-0.227250362890276,6.45268625633124,
3.53107252428385));
#14358=CARTESIAN_POINT('Ctrl Pts',(-0.00982453983942397,6.43239259089565,
3.63631313688574));
#14359=CARTESIAN_POINT('Ctrl Pts',(0.119224416062016,6.414995879623,3.79796488057796));
#14360=CARTESIAN_POINT('Ctrl Pts',(0.161414220224748,6.39904954972701,3.98302626625864));
#14361=CARTESIAN_POINT('Ctrl Pts',(0.132781651753175,6.38455548538367,4.15109736344141));
#14362=CARTESIAN_POINT('Ctrl Pts',(0.058591217696994,6.37151403493753,4.28547086198332));
#14363=CARTESIAN_POINT('Ctrl Pts',(-0.0558362639783319,6.35847699034469,
4.38747481451575));
#14364=CARTESIAN_POINT('Ctrl Pts',(-0.244624220570673,6.34110173177432,
4.46620946091905));
#14365=CARTESIAN_POINT('Ctrl Pts',(-0.509258386493358,6.31939963958705,
4.43663450707748));
#14366=CARTESIAN_POINT('Ctrl Pts',(-0.735030443095589,6.29339375292805,
4.21063569075453));
#14367=CARTESIAN_POINT('Ctrl Pts',(-0.770492148406669,6.2674338232997,3.89395438143295));
#14368=CARTESIAN_POINT('Ctrl Pts',(-0.601210048531917,6.24152902186401,
3.62457992816658));
#14369=CARTESIAN_POINT('Ctrl Pts',(-0.351688619951789,6.21999512440529,
3.53770552245775));
#14370=CARTESIAN_POINT('Ctrl Pts',(-0.152299417857812,6.20280445728418,
3.57207084012085));
#14371=CARTESIAN_POINT('Ctrl Pts',(-0.00495835013055459,6.18850033974624,
3.65330634586973));
#14372=CARTESIAN_POINT('Ctrl Pts',(0.111522803781729,6.17279483671223,3.79940640678234));
#14373=CARTESIAN_POINT('Ctrl Pts',(0.156701474788417,6.15570021231953,3.99770463755195));
#14374=CARTESIAN_POINT('Ctrl Pts',(0.115262604711903,6.14006777305336,4.17897821875209));
#14375=CARTESIAN_POINT('Ctrl Pts',(0.0185932180471106,6.12588811043834,
4.31497113433199));
#14376=CARTESIAN_POINT('Ctrl Pts',(-0.103590553659916,6.11315178814851,
4.4016989608744));
#14377=CARTESIAN_POINT('Ctrl Pts',(-0.247293954733903,6.1004417858412,4.44304193852122));
#14378=CARTESIAN_POINT('Ctrl Pts',(-0.412869049658234,6.08634982725544,
4.43379507168706));
#14379=CARTESIAN_POINT('Ctrl Pts',(-0.578482300908516,6.07088880084204,
4.3539190346138));
#14380=CARTESIAN_POINT('Ctrl Pts',(-0.703246723757797,6.05407432044984,
4.19753682982269));
#14381=CARTESIAN_POINT('Ctrl Pts',(-0.747469580607062,6.03731392465469,
4.00314057125818));
#14382=CARTESIAN_POINT('Ctrl Pts',(-0.703238625925696,6.02060951959296,
3.80940575329504));
#14383=CARTESIAN_POINT('Ctrl Pts',(-0.579634776479789,6.00396293095479,
3.65467865258803));
#14384=CARTESIAN_POINT('Ctrl Pts',(-0.431500759601328,5.99014040360805,
3.58338254073736));
#14385=CARTESIAN_POINT('Ctrl Pts',(-0.303561319206374,5.97911298339926,
3.56906449106088));
#14386=CARTESIAN_POINT('Ctrl Pts',(-0.207808748835976,5.97085791464426,
3.57983145987356));
#14387=CARTESIAN_POINT('Ctrl Pts',(-0.117044922248722,5.96261853714979,
3.6116348383249));
#14388=CARTESIAN_POINT('Ctrl Pts',(-0.00861997369778145,5.95165386736835,
3.67968231581426));
#14389=CARTESIAN_POINT('Ctrl Pts',(0.0926329081004657,5.93798817658918,
3.80681756846826));
#14390=CARTESIAN_POINT('Ctrl Pts',(0.135870644163702,5.92165495155963,3.99626375633351));
#14391=CARTESIAN_POINT('Ctrl Pts',(0.0926387969430078,5.90538860209907,
4.18487776410349));
#14392=CARTESIAN_POINT('Ctrl Pts',(-0.0175125738479973,5.89054016294629,
4.32293582509909));
#14393=CARTESIAN_POINT('Ctrl Pts',(-0.156061008534171,5.87709197920747,
4.39936287338782));
#14394=CARTESIAN_POINT('Ctrl Pts',(-0.296018497756522,5.86502791432804,
4.42315611503599));
#14395=CARTESIAN_POINT('Ctrl Pts',(-0.435406476921251,5.8530035361086,4.39932451423293));
#14396=CARTESIAN_POINT('Ctrl Pts',(-0.600212844195293,5.83702437044493,
4.30861645270809));
#14397=CARTESIAN_POINT('Ctrl Pts',(-0.729945333339283,5.81715142573852,
4.10216892170714));
#14398=CARTESIAN_POINT('Ctrl Pts',(-0.696976009348358,5.7934671926544,3.81306008549607));
#14399=CARTESIAN_POINT('Ctrl Pts',(-0.492652698548329,5.76994854996481,
3.60918617550531));
#14400=CARTESIAN_POINT('Ctrl Pts',(-0.207515825799976,5.74659510021081,
3.57736699868709));
#14401=CARTESIAN_POINT('Ctrl Pts',(-0.00714719245692835,5.72727465695078,
3.70390131122158));
#14402=CARTESIAN_POINT('Ctrl Pts',(0.0800330609517386,5.71189866882786,
3.86253474741929));
#14403=CARTESIAN_POINT('Ctrl Pts',(0.0951821641861108,5.70424160396714,
3.95121652410011));
#14404=CARTESIAN_POINT('Ctrl Pts',(0.0951881709252366,5.70041484319491,
3.99573871784903));
#14405=CARTESIAN_POINT('Origin',(0.1,5.75,4.));
#14406=CARTESIAN_POINT('Origin',(0.1,5.75,4.));
#14407=CARTESIAN_POINT('Origin',(0.1,7.05,4.));
#16962=UNCERTAINTY_MEASURE_WITH_UNIT(LENGTH_MEASURE(0.001),#17047,
'DISTANCE_ACCURACY_VALUE',
'Maximum model space distance between geometric entities at asserted c
onnectivities');
#16993=UNCERTAINTY_MEASURE_WITH_UNIT(LENGTH_MEASURE(0.001),#17047,
'DISTANCE_ACCURACY_VALUE',
'Maximum model space distance between geometric entities at asserted c
onnectivities');
#17015=(
GEOMETRIC_REPRESENTATION_CONTEXT(3)
GLOBAL_UNCERTAINTY_ASSIGNED_CONTEXT((#16962))
GLOBAL_UNIT_ASSIGNED_CONTEXT((#17047,#17049,#17050))
REPRESENTATION_CONTEXT('','3D')
);
#17046=(
GEOMETRIC_REPRESENTATION_CONTEXT(3)
GLOBAL_UNCERTAINTY_ASSIGNED_CONTEXT((#16993))
GLOBAL_UNIT_ASSIGNED_CONTEXT((#17047,#17049,#17050))
REPRESENTATION_CONTEXT('','3D')
);
#17047=(
LENGTH_UNIT()
NAMED_UNIT(*)
SI_UNIT(.CENTI.,.METRE.)
);
#17049=(
NAMED_UNIT(*)
PLANE_ANGLE_UNIT()
SI_UNIT($,.RADIAN.)
);
#17050=(
NAMED_UNIT(*)
SI_UNIT($,.STERADIAN.)
SOLID_ANGLE_UNIT()
);
#17072=SHAPE_DEFINITION_REPRESENTATION(#17124,#17279);
#17124=PRODUCT_DEFINITION_SHAPE('',$,#17332);
#17279=SHAPE_REPRESENTATION('',(#9213),#17015);
#17310=PRODUCT_DEFINITION_CONTEXT('part definition',#17468,'design');
#17332=PRODUCT_DEFINITION('Preload spring','Preload spring',#17384,#17310);
#17384=PRODUCT_DEFINITION_FORMATION('',$,#17491);
#17468=APPLICATION_CONTEXT(
'Core Data for Automotive Mechanical Design Process');
#17469=PRODUCT_CONTEXT('part definition',#17468,'mechanical');
#17491=PRODUCT('Preload spring','Preload spring','Preload spring',(#17469));
#17585=COLOUR_RGB('Grey',0.48,0.52,0.57);
#17586=FILL_AREA_STYLE_COLOUR('',#17585);
#17587=FILL_AREA_STYLE('',(#17586));
#17588=SURFACE_STYLE_FILL_AREA(#17587);
#17589=SURFACE_SIDE_STYLE('',(#17588));
#17590=SURFACE_STYLE_USAGE(.BOTH.,#17589);
#17591=PRESENTATION_STYLE_ASSIGNMENT((#17590));
ENDSEC;
END-ISO-10303-21;
